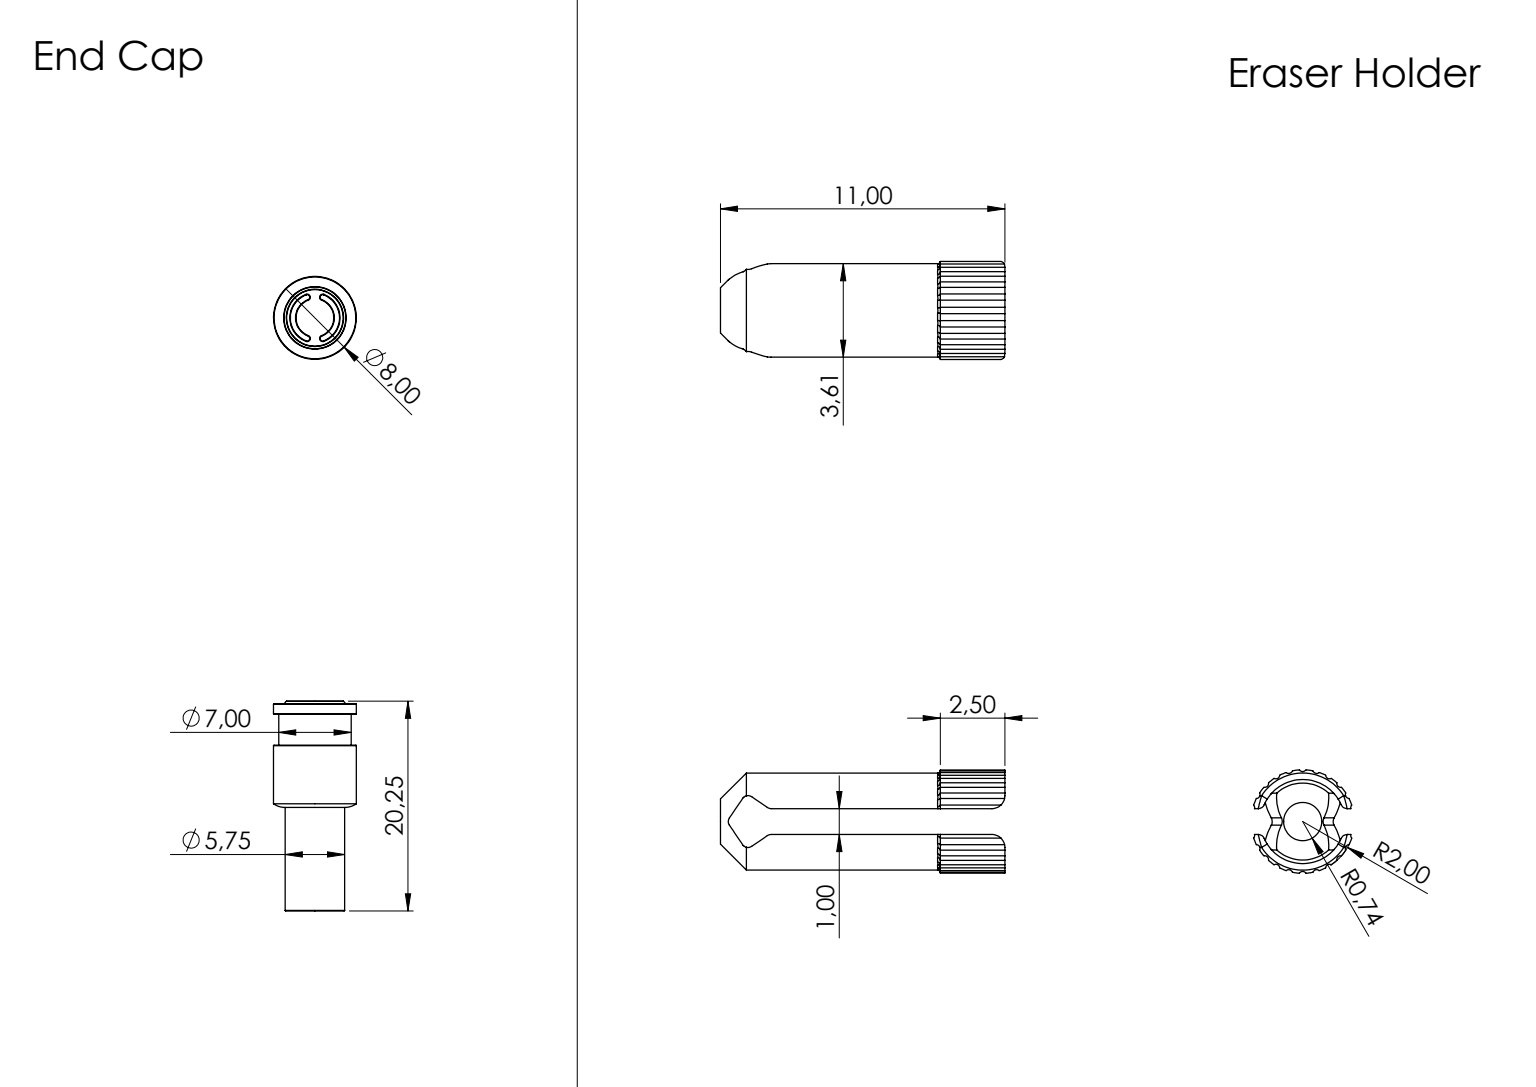
ISO-10303-21;
HEADER;
FILE_DESCRIPTION (('STEP AP214'),
    '1' );
FILE_NAME ('End Cap.step',
    '2026-10-06T14:00:01',
    ( '' ),
    ( '' ),
    'SwSTEP 2.0',
    'SolidWorks 2020',
    '' );
FILE_SCHEMA (( 'AUTOMOTIVE_DESIGN' ));
ENDSEC;

DATA;
#24=ORIENTED_EDGE ( 'NONE', *, *, #28945, .F. ) ;
#26=FACE_OUTER_BOUND ( 'NONE', #14344, .T. ) ;
#31=ORIENTED_EDGE ( 'NONE', *, *, #27047, .T. ) ;
#73=CARTESIAN_POINT ( 'NONE',  ( 63.50000000000004263, 0.7500000000000000000, 1.988246715072691018 ) ) ;
#80=DIRECTION ( 'NONE',  ( -1.000000000000000000, 0.000000000000000000, 1.047444401652940007E-14 ) ) ;
#85=( NAMED_UNIT ( * ) SI_UNIT ( $, .STERADIAN. ) SOLID_ANGLE_UNIT ( ) );
#109=EDGE_LOOP ( 'NONE', ( #31265, #1632, #31131, #2632 ) ) ;
#130=ORIENTED_EDGE ( 'NONE', *, *, #8388, .T. ) ;
#171=VERTEX_POINT ( 'NONE', #25293 ) ;
#187=FACE_OUTER_BOUND ( 'NONE', #28111, .T. ) ;
#235=ORIENTED_EDGE ( 'NONE', *, *, #4200, .F. ) ;
#258=CIRCLE ( 'NONE', #12381, 0.2999999999999999334 ) ;
#277=TOROIDAL_SURFACE ( 'NONE', #6855, 3.950000000000000178, 0.05000000000000000278 ) ;
#289=FACE_OUTER_BOUND ( 'NONE', #17501, .T. ) ;
#305=CIRCLE ( 'NONE', #30133, 0.05000000000000014849 ) ;
#318=AXIS2_PLACEMENT_3D ( 'NONE', #9279, #4194, #20999 ) ;
#319=ORIENTED_EDGE ( 'NONE', *, *, #23903, .T. ) ;
#326=ORIENTED_EDGE ( 'NONE', *, *, #1422, .T. ) ;
#340=CIRCLE ( 'NONE', #30668, 0.05000000000000007216 ) ;
#342=PLANE ( 'NONE',  #13632 ) ;
#352=DIRECTION ( 'NONE',  ( -1.000000000000000000, -0.000000000000000000, 1.047444401652940007E-14 ) ) ;
#365=AXIS2_PLACEMENT_3D ( 'NONE', #25779, #23413, #7408 ) ;
#369=ORIENTED_EDGE ( 'NONE', *, *, #19982, .T. ) ;
#372=ORIENTED_EDGE ( 'NONE', *, *, #29152, .T. ) ;
#391=( NAMED_UNIT ( * ) PLANE_ANGLE_UNIT ( ) SI_UNIT ( $, .RADIAN. ) );
#430=ORIENTED_EDGE ( 'NONE', *, *, #6181, .F. ) ;
#439=CARTESIAN_POINT ( 'NONE',  ( 69.20000000000005969, -0.7500000000000000000, 1.988246715072633508 ) ) ;
#454=DIRECTION ( 'NONE',  ( -1.000000000000000000, 0.000000000000000000, 1.047444401652940007E-14 ) ) ;
#460=EDGE_CURVE ( 'NONE', #25198, #24785, #24329, .T. ) ;
#474=ORIENTED_EDGE ( 'NONE', *, *, #7320, .T. ) ;
#479=DIRECTION ( 'NONE',  ( 1.000000000000000000, -0.000000000000000000, -1.047444401652940007E-14 ) ) ;
#486=APPLICATION_CONTEXT ( 'automotive_design' ) ;
#491=TOROIDAL_SURFACE ( 'NONE', #10107, 2.674999999999998934, 0.05000000000000000278 ) ;
#501=EDGE_CURVE ( 'NONE', #21780, #20962, #6621, .T. ) ;
#506=DIRECTION ( 'NONE',  ( 0.000000000000000000, -0.3529411764705882026, -0.9356455129756979794 ) ) ;
#512=PLANE ( 'NONE',  #27168 ) ;
#523=AXIS2_PLACEMENT_3D ( 'NONE', #6717, #4335, #11637 ) ;
#537=DIRECTION ( 'NONE',  ( 0.000000000000000000, 0.000000000000000000, -1.000000000000000000 ) ) ;
#590=VERTEX_POINT ( 'NONE', #30867 ) ;
#592=DIRECTION ( 'NONE',  ( 1.000000000000000000, -0.000000000000000000, -1.047444401652940007E-14 ) ) ;
#596=VERTEX_POINT ( 'NONE', #23754 ) ;
#602=EDGE_CURVE ( 'NONE', #9917, #10580, #19823, .T. ) ;
#617=FACE_OUTER_BOUND ( 'NONE', #26372, .T. ) ;
#662=DIRECTION ( 'NONE',  ( -1.000000000000000000, 0.000000000000000000, 1.047444401652940007E-14 ) ) ;
#666=ORIENTED_EDGE ( 'NONE', *, *, #5798, .T. ) ;
#670=EDGE_CURVE ( 'NONE', #23530, #30383, #28927, .T. ) ;
#679=DIRECTION ( 'NONE',  ( 1.000000000000000000, 0.000000000000000000, -1.047444401652940007E-14 ) ) ;
#690=DIRECTION ( 'NONE',  ( -1.000000000000000000, 0.000000000000000000, 1.047444401652940007E-14 ) ) ;
#696=ADVANCED_FACE ( 'NONE', ( #29416 ), #18309, .T. ) ;
#723=LINE ( 'NONE', #10382, #22147 ) ;
#738=EDGE_CURVE ( 'NONE', #5843, #8754, #4762, .T. ) ;
#757=CARTESIAN_POINT ( 'NONE',  ( 68.00000000000001421, 1.401298464324817071E-42, -7.122621931239992550E-13 ) ) ;
#763=VECTOR ( 'NONE', #13667, 1000.000000000000114 ) ;
#776=DIRECTION ( 'NONE',  ( 1.000000000000000000, -0.000000000000000000, -1.047444401652940007E-14 ) ) ;
#799=DIRECTION ( 'NONE',  ( 1.000000000000000000, 0.000000000000000000, -1.047444401652940007E-14 ) ) ;
#808=DIRECTION ( 'NONE',  ( 1.000000000000000000, -0.000000000000000000, -1.047444401652940007E-14 ) ) ;
#815=CIRCLE ( 'NONE', #18531, 0.2999999999999999334 ) ;
#824=DIRECTION ( 'NONE',  ( -1.000000000000000000, 0.000000000000000000, 1.047444401652940007E-14 ) ) ;
#859=EDGE_CURVE ( 'NONE', #27662, #23750, #12840, .T. ) ;
#865=VERTEX_POINT ( 'NONE', #10878 ) ;
#868=CLOSED_SHELL ( 'NONE', ( #3607, #31285, #19814, #2896, #11313, #1933, #16606, #2566, #11194, #9119, #8437, #4942, #20881, #10226, #9824, #19849, #13450, #13335, #9869, #14567, #23249, #23818, #19671, #16010, #18689, #8050, #28313, #23742, #25301, #4603, #23913, #2405, #3250, #16375, #22683, #11024, #14689, #29311, #10151, #2320, #31083, #28868, #9802, #29845, #22522, #28501, #27572, #16956, #21743, #3102, #20819, #24145, #21081, #696, #22329, #7299, #2322, #17235, #15972, #26956, #25336, #8923, #24762, #17568 ) ) ;
#899=TOROIDAL_SURFACE ( 'NONE', #1389, 1.824999999999999956, 0.05000000000000000278 ) ;
#913=EDGE_LOOP ( 'NONE', ( #29372, #10833, #15778, #13748, #18804, #24361, #21663, #28963, #6278, #30255, #1776, #13627, #28648, #7508, #21353, #15239 ) ) ;
#914=DIRECTION ( 'NONE',  ( -1.000000000000000000, 0.000000000000000000, 1.047444401652940007E-14 ) ) ;
#924=EDGE_LOOP ( 'NONE', ( #13849, #2269, #25709, #4752 ) ) ;
#937=TOROIDAL_SURFACE ( 'NONE', #5490, 3.950000000000000178, 0.05000000000000000278 ) ;
#1025=ORIENTED_EDGE ( 'NONE', *, *, #13535, .T. ) ;
#1027=CIRCLE ( 'NONE', #6586, 0.2999999999999999334 ) ;
#1078=EDGE_CURVE ( 'NONE', #25198, #6138, #25891, .T. ) ;
#1094=AXIS2_PLACEMENT_3D ( 'NONE', #17029, #80, #10049 ) ;
#1102=CARTESIAN_POINT ( 'NONE',  ( 67.99999999999998579, 1.401298464324817071E-42, -2.375000000000710543 ) ) ;
#1173=CARTESIAN_POINT ( 'NONE',  ( 68.00000000000000000, -0.6617647058823529216, -1.754335336830145975 ) ) ;
#1176=EDGE_LOOP ( 'NONE', ( #16382, #26534, #25910, #24778 ) ) ;
#1254=CARTESIAN_POINT ( 'NONE',  ( 68.05000000000006821, 4.898587196589419731E-16, 3.999999999999287237 ) ) ;
#1283=ORIENTED_EDGE ( 'NONE', *, *, #4003, .T. ) ;
#1296=AXIS2_PLACEMENT_3D ( 'NONE', #22942, #10594, #8211 ) ;
#1322=VECTOR ( 'NONE', #690, 1000.000000000000000 ) ;
#1330=ORIENTED_EDGE ( 'NONE', *, *, #14511, .F. ) ;
#1340=CARTESIAN_POINT ( 'NONE',  ( 60.67929986713514978, 1.401298464324817071E-42, -6.355819294205068152E-13 ) ) ;
#1361=TOROIDAL_SURFACE ( 'NONE', #10968, 0.3000000000000000444, 0.05000000000000000278 ) ;
#1385=VECTOR ( 'NONE', #24043, 1000.000000000000000 ) ;
#1389=AXIS2_PLACEMENT_3D ( 'NONE', #19677, #29454, #22353 ) ;
#1422=EDGE_CURVE ( 'NONE', #14417, #27508, #12555, .T. ) ;
#1434=EDGE_CURVE ( 'NONE', #12273, #27518, #6793, .T. ) ;
#1444=EDGE_LOOP ( 'NONE', ( #5295, #15394 ) ) ;
#1450=DIRECTION ( 'NONE',  ( 1.000000000000000000, -0.000000000000000000, -1.047444401652940007E-14 ) ) ;
#1517=EDGE_LOOP ( 'NONE', ( #10786, #26947 ) ) ;
#1554=DIRECTION ( 'NONE',  ( 0.000000000000000000, 0.000000000000000000, 1.000000000000000000 ) ) ;
#1566=DIRECTION ( 'NONE',  ( 1.000000000000000000, -0.000000000000000000, -1.047444401652940007E-14 ) ) ;
#1585=CARTESIAN_POINT ( 'NONE',  ( 67.99999999999998579, 3.214697847761800597E-16, -2.625000000000710987 ) ) ;
#1614=CARTESIAN_POINT ( 'NONE',  ( 63.50000000000000000, 0.7500000000000000000, -2.238246715074021953 ) ) ;
#1632=ORIENTED_EDGE ( 'NONE', *, *, #29506, .T. ) ;
#1669=EDGE_CURVE ( 'NONE', #12243, #22848, #26520, .T. ) ;
#1673=ORIENTED_EDGE ( 'NONE', *, *, #1078, .F. ) ;
#1683=CARTESIAN_POINT ( 'NONE',  ( 49.00000000000004263, -0.6617647058823530326, 1.754335336828920511 ) ) ;
#1692=VERTEX_POINT ( 'NONE', #27979 ) ;
#1728=DIRECTION ( 'NONE',  ( 1.040834085586084257E-14, 0.000000000000000000, 1.000000000000000000 ) ) ;
#1729=DIRECTION ( 'NONE',  ( -1.000000000000000000, -0.000000000000000000, 1.047444401652940007E-14 ) ) ;
#1752=VERTEX_POINT ( 'NONE', #10881 ) ;
#1766=EDGE_CURVE ( 'NONE', #1752, #14189, #12854, .T. ) ;
#1770=FACE_OUTER_BOUND ( 'NONE', #25402, .T. ) ;
#1775=DIRECTION ( 'NONE',  ( 0.000000000000000000, 0.000000000000000000, -1.000000000000000000 ) ) ;
#1776=ORIENTED_EDGE ( 'NONE', *, *, #6848, .T. ) ;
#1779=PLANE ( 'NONE',  #27597 ) ;
#1785=VERTEX_POINT ( 'NONE', #1980 ) ;
#1789=CARTESIAN_POINT ( 'NONE',  ( 69.24999999999998579, 3.823533025773894613E-16, -2.750000000000725198 ) ) ;
#1793=CARTESIAN_POINT ( 'NONE',  ( 68.00000000000004263, 0.8382352941176474115, 2.222158093316569438 ) ) ;
#1811=EDGE_CURVE ( 'NONE', #13465, #25040, #31059, .T. ) ;
#1853=CARTESIAN_POINT ( 'NONE',  ( 69.25000000000004263, -0.7500000000000000000, 1.988246715072630844 ) ) ;
#1869=CARTESIAN_POINT ( 'NONE',  ( 49.00000000000002132, 1.401298464324817071E-42, -5.132477568099407673E-13 ) ) ;
#1890=ORIENTED_EDGE ( 'NONE', *, *, #27079, .T. ) ;
#1912=CARTESIAN_POINT ( 'NONE',  ( 65.00000000000007105, 1.401298464324817071E-42, 3.499999999999319211 ) ) ;
#1933=ADVANCED_FACE ( 'NONE', ( #21468 ), #23872, .T. ) ;
#1963=EDGE_LOOP ( 'NONE', ( #10035, #26095, #29334, #18935, #7350, #21515, #2912 ) ) ;
#1966=EDGE_LOOP ( 'NONE', ( #11467, #21378, #11264, #28038 ) ) ;
#1976=VERTEX_POINT ( 'NONE', #17476 ) ;
#1980=CARTESIAN_POINT ( 'NONE',  ( 69.00000000000000000, 4.155057991226904698E-16, -3.020710678119368886 ) ) ;
#1984=CARTESIAN_POINT ( 'NONE',  ( 68.00000000000000000, 0.5000000000000000000, -1.988246715074070581 ) ) ;
#2001=DIRECTION ( 'NONE',  ( 1.000000000000000000, 0.000000000000000000, -1.047444401652940007E-14 ) ) ;
#2052=EDGE_CURVE ( 'NONE', #14020, #27339, #18813, .T. ) ;
#2071=CARTESIAN_POINT ( 'NONE',  ( 69.20000000000001705, 0.6617647058823536987, -1.754335336830159076 ) ) ;
#2089=DIRECTION ( 'NONE',  ( -1.047444401652940007E-14, 0.000000000000000000, -1.000000000000000000 ) ) ;
#2133=FACE_OUTER_BOUND ( 'NONE', #19427, .T. ) ;
#2155=EDGE_CURVE ( 'NONE', #20739, #26219, #22857, .T. ) ;
#2160=ORIENTED_EDGE ( 'NONE', *, *, #24446, .T. ) ;
#2166=DIRECTION ( 'NONE',  ( 1.000000000000000000, 0.000000000000000000, -1.047444401652940007E-14 ) ) ;
#2205=CARTESIAN_POINT ( 'NONE',  ( 49.00000000000000000, -0.6617647058823530326, -1.754335336829947023 ) ) ;
#2229=ORIENTED_EDGE ( 'NONE', *, *, #25840, .T. ) ;
#2256=DIRECTION ( 'NONE',  ( 1.000000000000000000, 0.000000000000000000, -1.047444401652940007E-14 ) ) ;
#2269=ORIENTED_EDGE ( 'NONE', *, *, #25539, .T. ) ;
#2275=DIRECTION ( 'NONE',  ( 1.000000000000000000, -0.000000000000000000, -1.047444401652940007E-14 ) ) ;
#2284=DIRECTION ( 'NONE',  ( -1.144559819201192819E-14, 0.000000000000000000, -1.000000000000000000 ) ) ;
#2296=DIRECTION ( 'NONE',  ( 1.047444401652940007E-14, 0.000000000000000000, 1.000000000000000000 ) ) ;
#2310=CARTESIAN_POINT ( 'NONE',  ( 69.20000000000001705, -0.7500000000000000000, -1.988246715074082793 ) ) ;
#2320=ADVANCED_FACE ( 'NONE', ( #26791 ), #10012, .F. ) ;
#2322=ADVANCED_FACE ( 'NONE', ( #16982 ), #491, .T. ) ;
#2327=DIRECTION ( 'NONE',  ( -1.000000000000000000, 0.000000000000000000, 1.047444401652940007E-14 ) ) ;
#2328=CIRCLE ( 'NONE', #6366, 3.500000000000000000 ) ;
#2329=CIRCLE ( 'NONE', #22049, 0.2500000000000002220 ) ;
#2343=ORIENTED_EDGE ( 'NONE', *, *, #19355, .F. ) ;
#2361=VECTOR ( 'NONE', #20954, 1000.000000000000000 ) ;
#2376=AXIS2_PLACEMENT_3D ( 'NONE', #4697, #2327, #21679 ) ;
#2377=TOROIDAL_SURFACE ( 'NONE', #10980, 0.3000000000000000444, 0.05000000000000000278 ) ;
#2390=CIRCLE ( 'NONE', #20103, 0.05000000000000012768 ) ;
#2405=ADVANCED_FACE ( 'NONE', ( #23799, #187, #22044 ), #342, .T. ) ;
#2482=DIRECTION ( 'NONE',  ( -1.047444401652940007E-14, 0.000000000000000000, -1.000000000000000000 ) ) ;
#2521=STYLED_ITEM ( 'NONE', ( #12068 ), #28934 ) ;
#2558=ORIENTED_EDGE ( 'NONE', *, *, #15305, .T. ) ;
#2565=SURFACE_STYLE_FILL_AREA ( #28995 ) ;
#2566=ADVANCED_FACE ( 'NONE', ( #11393 ), #11623, .T. ) ;
#2568=DIRECTION ( 'NONE',  ( -1.000000000000000000, 0.000000000000000000, 1.047444401652940007E-14 ) ) ;
#2591=DIRECTION ( 'NONE',  ( 1.047444401652940007E-14, 0.000000000000000000, 1.000000000000000000 ) ) ;
#2597=ORIENTED_EDGE ( 'NONE', *, *, #12546, .T. ) ;
#2632=ORIENTED_EDGE ( 'NONE', *, *, #11598, .F. ) ;
#2633=DIRECTION ( 'NONE',  ( 9.654113257610060303E-15, 0.000000000000000000, 1.000000000000000000 ) ) ;
#2689=DIRECTION ( 'NONE',  ( 0.000000000000000000, 0.000000000000000000, -1.000000000000000000 ) ) ;
#2696=CIRCLE ( 'NONE', #21934, 0.05000000000000012768 ) ;
#2699=CIRCLE ( 'NONE', #20918, 3.950000000000000178 ) ;
#2708=CARTESIAN_POINT ( 'NONE',  ( 69.25000000000000000, -0.7500000000000000000, -1.988246715074083681 ) ) ;
#2716=CIRCLE ( 'NONE', #6762, 2.374999999999998668 ) ;
#2745=VERTEX_POINT ( 'NONE', #14391 ) ;
#2748=LINE ( 'NONE', #17317, #16749 ) ;
#2761=EDGE_CURVE ( 'NONE', #21492, #16699, #6541, .T. ) ;
#2763=ORIENTED_EDGE ( 'NONE', *, *, #24226, .F. ) ;
#2779=AXIS2_PLACEMENT_3D ( 'NONE', #22887, #11146, #6100 ) ;
#2788=DIRECTION ( 'NONE',  ( -1.000000000000000000, 0.000000000000000000, 1.047444401652940007E-14 ) ) ;
#2792=CARTESIAN_POINT ( 'NONE',  ( 68.00000000000004263, 0.5000000000000000000, 1.988246715072646387 ) ) ;
#2797=AXIS2_PLACEMENT_3D ( 'NONE', #16721, #25731, #14318 ) ;
#2798=EDGE_LOOP ( 'NONE', ( #5175, #12651, #13298, #19894 ) ) ;
#2799=DIRECTION ( 'NONE',  ( 1.040834085586084257E-14, 0.000000000000000000, 1.000000000000000000 ) ) ;
#2811=DIRECTION ( 'NONE',  ( -1.000000000000000000, -0.000000000000000000, 1.047444401652940007E-14 ) ) ;
#2815=AXIS2_PLACEMENT_3D ( 'NONE', #16284, #25927, #4230 ) ;
#2873=CIRCLE ( 'NONE', #17554, 2.985355339059319046 ) ;
#2896=ADVANCED_FACE ( 'NONE', ( #3432 ), #10591, .F. ) ;
#2911=DIRECTION ( 'NONE',  ( -1.000000000000000000, -0.000000000000000000, 1.047444401652940007E-14 ) ) ;
#2912=ORIENTED_EDGE ( 'NONE', *, *, #24728, .T. ) ;
#2922=SURFACE_STYLE_FILL_AREA ( #16873 ) ;
#2956=PRODUCT_DEFINITION ( 'UNKNOWN', '', #17169, #15507 ) ;
#2979=LINE ( 'NONE', #9792, #28702 ) ;
#2982=DIRECTION ( 'NONE',  ( 0.000000000000000000, 0.000000000000000000, -1.000000000000000000 ) ) ;
#3000=CARTESIAN_POINT ( 'NONE',  ( 49.00000000000004974, 1.401298464324817071E-42, 2.824999999999485922 ) ) ;
#3035=CARTESIAN_POINT ( 'NONE',  ( 69.25000000000001421, 4.557543281186736018E-17, -7.253552481446610839E-13 ) ) ;
#3049=DIRECTION ( 'NONE',  ( 0.000000000000000000, -1.224646799147343593E-16, 1.000000000000000000 ) ) ;
#3050=CARTESIAN_POINT ( 'NONE',  ( 68.00000000000002842, 1.401298464324817071E-42, -7.122621931239993559E-13 ) ) ;
#3064=VERTEX_POINT ( 'NONE', #13827 ) ;
#3094=ORIENTED_EDGE ( 'NONE', *, *, #7320, .F. ) ;
#3102=ADVANCED_FACE ( 'NONE', ( #16561 ), #9433, .T. ) ;
#3117=EDGE_CURVE ( 'NONE', #24431, #23786, #25591, .T. ) ;
#3223=EDGE_CURVE ( 'NONE', #171, #9260, #10953, .T. ) ;
#3232=AXIS2_PLACEMENT_3D ( 'NONE', #3050, #824, #8112 ) ;
#3250=ADVANCED_FACE ( 'NONE', ( #5739 ), #28634, .T. ) ;
#3256=AXIS2_PLACEMENT_3D ( 'NONE', #9828, #19494, #5079 ) ;
#3264=AXIS2_PLACEMENT_3D ( 'NONE', #8768, #18933, #21165 ) ;
#3265=LINE ( 'NONE', #22761, #28622 ) ;
#3270=AXIS2_PLACEMENT_3D ( 'NONE', #13221, #20700, #30471 ) ;
#3274=DIRECTION ( 'NONE',  ( -1.047444401652940007E-14, 0.000000000000000000, -1.000000000000000000 ) ) ;
#3276=CARTESIAN_POINT ( 'NONE',  ( 69.20000000000001705, -0.5000000000000000000, -1.988246715074081017 ) ) ;
#3295=CARTESIAN_POINT ( 'NONE',  ( 65.00000000000002842, 1.401298464324817071E-42, -6.808388610744111684E-13 ) ) ;
#3304=CIRCLE ( 'NONE', #9890, 3.020710678118645909 ) ;
#3317=CIRCLE ( 'NONE', #2815, 4.000000000000000000 ) ;
#3382=VECTOR ( 'NONE', #15294, 1000.000000000000000 ) ;
#3387=DIRECTION ( 'NONE',  ( 1.047444401652940007E-14, 0.000000000000000000, 1.000000000000000000 ) ) ;
#3432=FACE_OUTER_BOUND ( 'NONE', #1176, .T. ) ;
#3433=CARTESIAN_POINT ( 'NONE',  ( 69.00000000000005684, 1.401298464324817071E-42, 3.949999999999278089 ) ) ;
#3442=CARTESIAN_POINT ( 'NONE',  ( 68.95000000000007390, 1.401298464324817071E-42, 3.949999999999278089 ) ) ;
#3506=DIRECTION ( 'NONE',  ( 1.000000000000000000, 0.000000000000000000, -1.047444401652940007E-14 ) ) ;
#3517=FACE_OUTER_BOUND ( 'NONE', #4297, .T. ) ;
#3522=DIRECTION ( 'NONE',  ( 1.168655815394902336E-14, 0.000000000000000000, 1.000000000000000000 ) ) ;
#3526=EDGE_LOOP ( 'NONE', ( #19588, #28740, #24, #29141 ) ) ;
#3530=DIRECTION ( 'NONE',  ( -3.198643159535995633E-15, -0.9356455129756995337, -0.3529411764705844834 ) ) ;
#3531=DIRECTION ( 'NONE',  ( 1.000000000000000000, 0.000000000000000000, -1.047444401652940007E-14 ) ) ;
#3543=DIRECTION ( 'NONE',  ( 1.000000000000000000, 0.000000000000000000, -8.673617379884989994E-15 ) ) ;
#3548=CARTESIAN_POINT ( 'NONE',  ( 49.05000000000002558, 1.401298464324817071E-42, -5.137714790107672405E-13 ) ) ;
#3607=ADVANCED_FACE ( 'NONE', ( #24484 ), #22978, .T. ) ;
#3713=ORIENTED_EDGE ( 'NONE', *, *, #27923, .F. ) ;
#3719=DIRECTION ( 'NONE',  ( -1.000000000000000000, 0.000000000000000000, 1.047444401652940007E-14 ) ) ;
#3738=ORIENTED_EDGE ( 'NONE', *, *, #8941, .F. ) ;
#3789=ORIENTED_EDGE ( 'NONE', *, *, #20362, .F. ) ;
#3797=CARTESIAN_POINT ( 'NONE',  ( 69.20000000000001705, 0.4500000000000000111, -1.988246715074080573 ) ) ;
#3811=DIRECTION ( 'NONE',  ( 1.000000000000000000, 0.000000000000000000, -1.047444401652940007E-14 ) ) ;
#3817=VERTEX_POINT ( 'NONE', #30595 ) ;
#3836=AXIS2_PLACEMENT_3D ( 'NONE', #5703, #8382, #22493 ) ;
#3844=EDGE_CURVE ( 'NONE', #14189, #1752, #2699, .T. ) ;
#3847=EDGE_CURVE ( 'NONE', #26053, #4809, #15343, .T. ) ;
#3856=VECTOR ( 'NONE', #15914, 1000.000000000000000 ) ;
#3869=AXIS2_PLACEMENT_3D ( 'NONE', #11567, #28818, #21242 ) ;
#3883=CIRCLE ( 'NONE', #21613, 0.2500000000000000000 ) ;
#3920=CIRCLE ( 'NONE', #27677, 1.874999999999998668 ) ;
#3988=ORIENTED_EDGE ( 'NONE', *, *, #18972, .F. ) ;
#4003=EDGE_CURVE ( 'NONE', #8546, #4409, #24941, .T. ) ;
#4006=DIRECTION ( 'NONE',  ( -1.040834085586084257E-14, 0.000000000000000000, -1.000000000000000000 ) ) ;
#4014=DIRECTION ( 'NONE',  ( 1.000000000000000000, -0.000000000000000000, -1.047444401652940007E-14 ) ) ;
#4016=ORIENTED_EDGE ( 'NONE', *, *, #22796, .F. ) ;
#4021=ORIENTED_EDGE ( 'NONE', *, *, #26922, .T. ) ;
#4023=LINE ( 'NONE', #1789, #763 ) ;
#4042=CIRCLE ( 'NONE', #19235, 0.05000000000000012768 ) ;
#4065=CARTESIAN_POINT ( 'NONE',  ( 58.99999999999999289, 4.286263797015737088E-16, -3.000000000000618172 ) ) ;
#4097=VERTEX_POINT ( 'NONE', #22985 ) ;
#4142=EDGE_CURVE ( 'NONE', #13465, #11082, #28489, .T. ) ;
#4158=CARTESIAN_POINT ( 'NONE',  ( 69.25000000000004263, -0.4500000000000000111, 1.988246715072632620 ) ) ;
#4175=CARTESIAN_POINT ( 'NONE',  ( 64.95000000000001705, 1.401298464324817071E-42, -6.803151388735846952E-13 ) ) ;
#4194=DIRECTION ( 'NONE',  ( 0.000000000000000000, -1.000000000000000000, -0.000000000000000000 ) ) ;
#4200=EDGE_CURVE ( 'NONE', #8754, #8529, #16324, .T. ) ;
#4230=DIRECTION ( 'NONE',  ( -1.040834085586084257E-14, 0.000000000000000000, -1.000000000000000000 ) ) ;
#4263=DIRECTION ( 'NONE',  ( 1.000000000000000000, 0.000000000000000000, -1.047444401652940007E-14 ) ) ;
#4297=EDGE_LOOP ( 'NONE', ( #27696, #15667, #12138, #14102 ) ) ;
#4314=CIRCLE ( 'NONE', #15443, 4.000000000000000000 ) ;
#4335=DIRECTION ( 'NONE',  ( -1.000000000000000000, 0.000000000000000000, 1.047444401652940007E-14 ) ) ;
#4339=ORIENTED_EDGE ( 'NONE', *, *, #3223, .T. ) ;
#4386=AXIS2_PLACEMENT_3D ( 'NONE', #20623, #10633, #30085 ) ;
#4409=VERTEX_POINT ( 'NONE', #14725 ) ;
#4451=EDGE_LOOP ( 'NONE', ( #20168, #369, #23422, #5115 ) ) ;
#4471=CARTESIAN_POINT ( 'NONE',  ( 65.00000000000002842, 1.401298464324817071E-42, -6.808388610744111684E-13 ) ) ;
#4472=CARTESIAN_POINT ( 'NONE',  ( 69.25000000000001421, 4.557543281186736018E-17, -7.253552481446610839E-13 ) ) ;
#4522=FACE_OUTER_BOUND ( 'NONE', #25805, .T. ) ;
#4554=DIRECTION ( 'NONE',  ( 1.000000000000000000, -0.000000000000000000, -1.047444401652940007E-14 ) ) ;
#4565=CARTESIAN_POINT ( 'NONE',  ( 63.50000000000002842, 1.401298464324817071E-42, -6.651271950496169736E-13 ) ) ;
#4566=VERTEX_POINT ( 'NONE', #7905 ) ;
#4579=CYLINDRICAL_SURFACE ( 'NONE', #25145, 4.000000000000000000 ) ;
#4595=DIRECTION ( 'NONE',  ( 0.000000000000000000, 0.000000000000000000, -1.000000000000000000 ) ) ;
#4603=ADVANCED_FACE ( 'NONE', ( #27697 ), #12797, .T. ) ;
#4641=AXIS2_PLACEMENT_3D ( 'NONE', #6535, #25844, #25994 ) ;
#4659=ORIENTED_EDGE ( 'NONE', *, *, #9443, .F. ) ;
#4681=DIRECTION ( 'NONE',  ( 1.000000000000000000, -0.000000000000000000, -1.047444401652940007E-14 ) ) ;
#4686=CARTESIAN_POINT ( 'NONE',  ( 69.25000000000001421, 1.401298464324817071E-42, -7.253552481446610839E-13 ) ) ;
#4697=CARTESIAN_POINT ( 'NONE',  ( 59.35000000000002984, 1.401298464324817071E-42, -6.216582523810200043E-13 ) ) ;
#4722=AXIS2_PLACEMENT_3D ( 'NONE', #17774, #30404, #22841 ) ;
#4752=ORIENTED_EDGE ( 'NONE', *, *, #29152, .F. ) ;
#4762=CIRCLE ( 'NONE', #19449, 2.624999999999998668 ) ;
#4778=AXIS2_PLACEMENT_3D ( 'NONE', #7989, #19867, #24604 ) ;
#4801=VERTEX_POINT ( 'NONE', #15636 ) ;
#4809=VERTEX_POINT ( 'NONE', #3276 ) ;
#4824=DIRECTION ( 'NONE',  ( -1.000000000000000000, 0.000000000000000000, 1.047444401652940007E-14 ) ) ;
#4825=CARTESIAN_POINT ( 'NONE',  ( 69.23535533905938166, 4.557543281186736018E-17, 2.764644660939941101 ) ) ;
#4840=DIRECTION ( 'NONE',  ( 1.000000000000000000, -0.000000000000000000, -1.047444401652940007E-14 ) ) ;
#4843=CARTESIAN_POINT ( 'NONE',  ( 68.00000000000000000, 0.7500000000000000000, -1.988246715074068582 ) ) ;
#4861=AXIS2_PLACEMENT_3D ( 'NONE', #18898, #23956, #16205 ) ;
#4880=CARTESIAN_POINT ( 'NONE',  ( 68.00000000000001421, 5.529431079676072613E-15, -7.122621931239992550E-13 ) ) ;
#4919=ORIENTED_EDGE ( 'NONE', *, *, #6181, .T. ) ;
#4928=( NAMED_UNIT ( * ) SI_UNIT ( $, .STERADIAN. ) SOLID_ANGLE_UNIT ( ) );
#4932=CIRCLE ( 'NONE', #25130, 2.874999999999999112 ) ;
#4942=ADVANCED_FACE ( 'NONE', ( #12268 ), #9903, .F. ) ;
#4959=FACE_OUTER_BOUND ( 'NONE', #16370, .T. ) ;
#4974=CARTESIAN_POINT ( 'NONE',  ( 65.00000000000007105, 4.867971026610729436E-16, 3.949999999999319389 ) ) ;
#4978=AXIS2_PLACEMENT_3D ( 'NONE', #73, #2275, #11940 ) ;
#4982=DIRECTION ( 'NONE',  ( 0.000000000000000000, 0.000000000000000000, -1.000000000000000000 ) ) ;
#5031=ORIENTED_EDGE ( 'NONE', *, *, #19144, .F. ) ;
#5051=CARTESIAN_POINT ( 'NONE',  ( 69.20000000000003126, 5.529431079676072613E-15, -7.248315259438346108E-13 ) ) ;
#5052=AXIS2_PLACEMENT_3D ( 'NONE', #23868, #7386, #19431 ) ;
#5079=DIRECTION ( 'NONE',  ( -7.401486830834377462E-15, 0.000000000000000000, -1.000000000000000000 ) ) ;
#5115=ORIENTED_EDGE ( 'NONE', *, *, #5759, .F. ) ;
#5127=ORIENTED_EDGE ( 'NONE', *, *, #24333, .F. ) ;
#5131=FACE_OUTER_BOUND ( 'NONE', #8472, .T. ) ;
#5138=CARTESIAN_POINT ( 'NONE',  ( 69.20000000000000284, -0.8558823529411765385, -2.268940368966790189 ) ) ;
#5175=ORIENTED_EDGE ( 'NONE', *, *, #18929, .F. ) ;
#5180=DIRECTION ( 'NONE',  ( 1.000000000000000000, 0.000000000000000000, -1.047444401652940007E-14 ) ) ;
#5218=CARTESIAN_POINT ( 'NONE',  ( 69.20000000000004547, 0.7500000000000000000, 1.988246715072631732 ) ) ;
#5226=ORIENTED_EDGE ( 'NONE', *, *, #18865, .F. ) ;
#5256=CARTESIAN_POINT ( 'NONE',  ( 68.94999999999998863, 4.837354856632045057E-16, -3.950000000000722711 ) ) ;
#5295=ORIENTED_EDGE ( 'NONE', *, *, #14044, .T. ) ;
#5306=CIRCLE ( 'NONE', #8845, 0.2999999999999999334 ) ;
#5348=CIRCLE ( 'NONE', #13423, 1.679509022399086948 ) ;
#5362=CIRCLE ( 'NONE', #24578, 0.05000000000000012768 ) ;
#5368=DIRECTION ( 'NONE',  ( -1.047444401652940007E-14, 0.000000000000000000, -1.000000000000000000 ) ) ;
#5381=AXIS2_PLACEMENT_3D ( 'NONE', #12530, #352, #26937 ) ;
#5385=DIRECTION ( 'NONE',  ( 1.168655815394902336E-14, 5.329070518200751394E-15, 1.000000000000000000 ) ) ;
#5411=DIRECTION ( 'NONE',  ( 1.047444401652940007E-14, 0.000000000000000000, 1.000000000000000000 ) ) ;
#5416=DIRECTION ( 'NONE',  ( -1.000000000000000000, 0.000000000000000000, 1.047444401652940007E-14 ) ) ;
#5436=AXIS2_PLACEMENT_3D ( 'NONE', #29883, #15788, #29727 ) ;
#5443=EDGE_LOOP ( 'NONE', ( #6142, #21561, #27785, #16734 ) ) ;
#5444=DIRECTION ( 'NONE',  ( 1.000000000000000000, -0.000000000000000000, -1.047444401652940007E-14 ) ) ;
#5456=CARTESIAN_POINT ( 'NONE',  ( 69.20000000000001705, -0.6441176470588234615, -1.707553061181373621 ) ) ;
#5465=ORIENTED_EDGE ( 'NONE', *, *, #5759, .T. ) ;
#5473=AXIS2_PLACEMENT_3D ( 'NONE', #13711, #30194, #10722 ) ;
#5490=AXIS2_PLACEMENT_3D ( 'NONE', #5911, #13312, #25370 ) ;
#5521=CARTESIAN_POINT ( 'NONE',  ( 69.20000000000003126, 1.401298464324817071E-42, -7.248315259438346108E-13 ) ) ;
#5589=CARTESIAN_POINT ( 'NONE',  ( 69.25000000000000000, -0.6441176470588234615, -1.707553061181374066 ) ) ;
#5640=LINE ( 'NONE', #17989, #3382 ) ;
#5646=LINE ( 'NONE', #23523, #3856 ) ;
#5672=LINE ( 'NONE', #24506, #9916 ) ;
#5703=CARTESIAN_POINT ( 'NONE',  ( 68.00000000000001421, 1.401298464324817071E-42, -7.122621931239992550E-13 ) ) ;
#5713=EDGE_CURVE ( 'NONE', #596, #25040, #2979, .T. ) ;
#5739=FACE_OUTER_BOUND ( 'NONE', #8033, .T. ) ;
#5759=EDGE_CURVE ( 'NONE', #25198, #27301, #19312, .T. ) ;
#5765=CARTESIAN_POINT ( 'NONE',  ( 59.00000000000006395, 4.898587196589412829E-16, 3.999999999999382716 ) ) ;
#5798=EDGE_CURVE ( 'NONE', #8746, #596, #3920, .T. ) ;
#5818=VERTEX_POINT ( 'NONE', #9952 ) ;
#5843=VERTEX_POINT ( 'NONE', #30025 ) ;
#5851=VECTOR ( 'NONE', #21513, 1000.000000000000000 ) ;
#5880=CIRCLE ( 'NONE', #9442, 0.2500000000000000000 ) ;
#5884=CARTESIAN_POINT ( 'NONE',  ( 69.25000000000000000, -0.7500000000000000000, -2.288246715074081283 ) ) ;
#5901=VERTEX_POINT ( 'NONE', #18014 ) ;
#5903=DIRECTION ( 'NONE',  ( -1.000000000000000000, -0.000000000000000000, 1.047444401652940007E-14 ) ) ;
#5911=CARTESIAN_POINT ( 'NONE',  ( 68.05000000000002558, 1.401298464324817071E-42, -7.127859153248258291E-13 ) ) ;
#5935=EDGE_CURVE ( 'NONE', #20739, #23786, #31228, .T. ) ;
#5937=ORIENTED_EDGE ( 'NONE', *, *, #18457, .T. ) ;
#5953=VERTEX_POINT ( 'NONE', #22780 ) ;
#5983=EDGE_LOOP ( 'NONE', ( #2229, #9730, #15226, #28249 ) ) ;
#5990=FACE_OUTER_BOUND ( 'NONE', #1966, .T. ) ;
#5993=DIRECTION ( 'NONE',  ( -9.654113257610060303E-15, 0.000000000000000000, -1.000000000000000000 ) ) ;
#6004=AXIS2_PLACEMENT_3D ( 'NONE', #21933, #27119, #10042 ) ;
#6014=ORIENTED_EDGE ( 'NONE', *, *, #19790, .T. ) ;
#6016=ORIENTED_EDGE ( 'NONE', *, *, #602, .F. ) ;
#6017=UNCERTAINTY_MEASURE_WITH_UNIT (LENGTH_MEASURE( 1.000000000000000082E-05 ), #6831, 'distance_accuracy_value', 'NONE');
#6023=EDGE_LOOP ( 'NONE', ( #3988, #12062, #15679, #11566, #29583, #12414, #7163, #22036 ) ) ;
#6049=DIRECTION ( 'NONE',  ( 1.003947306782822575E-14, 0.000000000000000000, 1.000000000000000000 ) ) ;
#6055=CARTESIAN_POINT ( 'NONE',  ( 68.95000000000003126, 1.401298464324817071E-42, -7.222129149397022450E-13 ) ) ;
#6062=FACE_OUTER_BOUND ( 'NONE', #18360, .T. ) ;
#6095=CARTESIAN_POINT ( 'NONE',  ( 64.99999999999998579, 4.286263797015736595E-16, -3.500000000000680789 ) ) ;
#6100=DIRECTION ( 'NONE',  ( 0.000000000000000000, 0.000000000000000000, -1.000000000000000000 ) ) ;
#6108=VERTEX_POINT ( 'NONE', #4065 ) ;
#6138=VERTEX_POINT ( 'NONE', #20864 ) ;
#6142=ORIENTED_EDGE ( 'NONE', *, *, #27708, .F. ) ;
#6158=EDGE_CURVE ( 'NONE', #9761, #29519, #8484, .T. ) ;
#6181=EDGE_CURVE ( 'NONE', #3817, #2745, #22155, .T. ) ;
#6204=EDGE_LOOP ( 'NONE', ( #235, #8965, #1890, #9902 ) ) ;
#6212=ORIENTED_EDGE ( 'NONE', *, *, #20691, .F. ) ;
#6241=CARTESIAN_POINT ( 'NONE',  ( 59.00000000000002132, 1.401298464324817071E-42, -6.179921969752347932E-13 ) ) ;
#6248=EDGE_LOOP ( 'NONE', ( #30369, #13520, #8307, #27484 ) ) ;
#6278=ORIENTED_EDGE ( 'NONE', *, *, #12527, .F. ) ;
#6290=EDGE_CURVE ( 'NONE', #9260, #18734, #19135, .T. ) ;
#6292=LINE ( 'NONE', #1683, #13720 ) ;
#6306=DIRECTION ( 'NONE',  ( 0.000000000000000000, 0.000000000000000000, -1.000000000000000000 ) ) ;
#6314=VERTEX_POINT ( 'NONE', #15606 ) ;
#6335=DIRECTION ( 'NONE',  ( 0.000000000000000000, 1.000000000000000000, -8.673617379884030739E-15 ) ) ;
#6347=DIRECTION ( 'NONE',  ( -9.654113257610060303E-15, 0.000000000000000000, -1.000000000000000000 ) ) ;
#6353=ORIENTED_EDGE ( 'NONE', *, *, #21694, .F. ) ;
#6366=AXIS2_PLACEMENT_3D ( 'NONE', #11355, #21044, #16429 ) ;
#6379=COLOUR_RGB ( '', 0.72549020, 0.75294118, 0.79215686) ;
#6392=AXIS2_PLACEMENT_3D ( 'NONE', #12568, #17654, #21801 ) ;
#6400=CIRCLE ( 'NONE', #318, 0.05000000000000012768 ) ;
#6405=CIRCLE ( 'NONE', #24108, 0.05000000000000014849 ) ;
#6416=CARTESIAN_POINT ( 'NONE',  ( 69.20000000000004547, -0.6617647058823530326, 1.754335336828708902 ) ) ;
#6435=CIRCLE ( 'NONE', #25111, 0.05000000000000012768 ) ;
#6436=ORIENTED_EDGE ( 'NONE', *, *, #9419, .F. ) ;
#6451=ORIENTED_EDGE ( 'NONE', *, *, #17555, .F. ) ;
#6461=DIRECTION ( 'NONE',  ( -1.000000000000000000, 0.000000000000000000, 1.047444401652940007E-14 ) ) ;
#6498=DIRECTION ( 'NONE',  ( 0.000000000000000000, 0.000000000000000000, -1.000000000000000000 ) ) ;
#6522=EDGE_LOOP ( 'NONE', ( #5031, #9393, #7409, #12142 ) ) ;
#6535=CARTESIAN_POINT ( 'NONE',  ( 68.00000000000004263, -0.7500000000000000000, 1.988246715072645943 ) ) ;
#6541=CIRCLE ( 'NONE', #12114, 2.374999999999998668 ) ;
#6557=DIRECTION ( 'NONE',  ( -1.047444401652940007E-14, 0.000000000000000000, -1.000000000000000000 ) ) ;
#6586=AXIS2_PLACEMENT_3D ( 'NONE', #12108, #13988, #7200 ) ;
#6621=CIRCLE ( 'NONE', #3836, 2.374999999999998668 ) ;
#6641=DIRECTION ( 'NONE',  ( 1.003947306782822575E-14, 0.000000000000000000, 1.000000000000000000 ) ) ;
#6687=DIRECTION ( 'NONE',  ( -1.282749433769087582E-30, 1.000000000000000000, -1.224646799147353207E-16 ) ) ;
#6710=CARTESIAN_POINT ( 'NONE',  ( 69.20000000000000284, -0.8382352941176473005, -2.222158093318006067 ) ) ;
#6717=CARTESIAN_POINT ( 'NONE',  ( 49.05000000000002558, 1.401298464324817071E-42, -5.137714790107672405E-13 ) ) ;
#6735=CARTESIAN_POINT ( 'NONE',  ( 67.99999999999997158, 1.401298464324817071E-42, -4.000000000000712319 ) ) ;
#6754=LINE ( 'NONE', #21671, #14045 ) ;
#6762=AXIS2_PLACEMENT_3D ( 'NONE', #10644, #662, #3522 ) ;
#6776=CARTESIAN_POINT ( 'NONE',  ( 68.00000000000000000, 0.8382352941176474115, -2.222158093317993632 ) ) ;
#6779=AXIS2_PLACEMENT_3D ( 'NONE', #12653, #20286, #10905 ) ;
#6793=CIRCLE ( 'NONE', #18945, 0.2999999999999999334 ) ;
#6796=CARTESIAN_POINT ( 'NONE',  ( 69.23535533905935324, 4.557543281186736018E-17, -7.252018534634969470E-13 ) ) ;
#6803=AXIS2_PLACEMENT_3D ( 'NONE', #19590, #4840, #9292 ) ;
#6814=DIRECTION ( 'NONE',  ( -1.000000000000000000, 0.000000000000000000, 1.047444401652940007E-14 ) ) ;
#6820=CIRCLE ( 'NONE', #24510, 0.2500000000000000000 ) ;
#6827=DIRECTION ( 'NONE',  ( -1.000000000000000000, -0.000000000000000000, 1.047444401652940007E-14 ) ) ;
#6831=( LENGTH_UNIT ( ) NAMED_UNIT ( * ) SI_UNIT ( .MILLI., .METRE. ) );
#6837=PRODUCT_DEFINITION_SHAPE ( 'NONE', 'NONE',  #2956 ) ;
#6842=DIRECTION ( 'NONE',  ( -1.000000000000000000, 0.000000000000000000, 1.047444401652940007E-14 ) ) ;
#6848=EDGE_CURVE ( 'NONE', #21838, #596, #7587, .T. ) ;
#6850=CYLINDRICAL_SURFACE ( 'NONE', #4861, 0.2500000000000002220 ) ;
#6855=AXIS2_PLACEMENT_3D ( 'NONE', #15685, #28009, #11227 ) ;
#6866=DIRECTION ( 'NONE',  ( 1.000000000000000000, -0.000000000000000000, -1.047444401652940007E-14 ) ) ;
#6873=AXIS2_PLACEMENT_3D ( 'NONE', #21591, #9560, #14430 ) ;
#6905=AXIS2_PLACEMENT_3D ( 'NONE', #31304, #4554, #21972 ) ;
#6927=CIRCLE ( 'NONE', #20581, 2.764644660940665855 ) ;
#6935=CARTESIAN_POINT ( 'NONE',  ( 68.00000000000001421, 1.401298464324817071E-42, -7.122621931239992550E-13 ) ) ;
#6970=DIRECTION ( 'NONE',  ( 1.037591611799212092E-14, 0.000000000000000000, 1.000000000000000000 ) ) ;
#7010=CARTESIAN_POINT ( 'NONE',  ( 69.00000000000001421, 4.557543281186736018E-17, -7.227366371405287181E-13 ) ) ;
#7015=DIRECTION ( 'NONE',  ( 1.000000000000000000, 0.000000000000000000, -1.047444401652940007E-14 ) ) ;
#7035=DIRECTION ( 'NONE',  ( -1.000000000000000000, 0.000000000000000000, 1.047444401652940007E-14 ) ) ;
#7062=CYLINDRICAL_SURFACE ( 'NONE', #17557, 4.000000000000000000 ) ;
#7092=DIRECTION ( 'NONE',  ( -1.000000000000000000, 0.000000000000000000, 1.047444401652940007E-14 ) ) ;
#7141=DIRECTION ( 'NONE',  ( 1.000000000000000000, -0.000000000000000000, -1.047444401652940007E-14 ) ) ;
#7160=( NAMED_UNIT ( * ) PLANE_ANGLE_UNIT ( ) SI_UNIT ( $, .RADIAN. ) );
#7163=ORIENTED_EDGE ( 'NONE', *, *, #19184, .T. ) ;
#7180=ORIENTED_EDGE ( 'NONE', *, *, #15305, .F. ) ;
#7199=DIRECTION ( 'NONE',  ( -1.000000000000000000, 0.000000000000000000, 1.047444401652940007E-14 ) ) ;
#7200=DIRECTION ( 'NONE',  ( 0.000000000000000000, 0.000000000000000000, -1.000000000000000000 ) ) ;
#7206=ORIENTED_EDGE ( 'NONE', *, *, #18972, .T. ) ;
#7209=EDGE_CURVE ( 'NONE', #31227, #21014, #22285, .T. ) ;
#7226=FACE_OUTER_BOUND ( 'NONE', #5983, .T. ) ;
#7232=EDGE_CURVE ( 'NONE', #4566, #6138, #20260, .T. ) ;
#7235=DIRECTION ( 'NONE',  ( 0.000000000000000000, -1.224646799147343593E-16, 1.000000000000000000 ) ) ;
#7238=DIRECTION ( 'NONE',  ( 1.000000000000000000, 0.000000000000000000, -1.047444401652940007E-14 ) ) ;
#7244=CARTESIAN_POINT ( 'NONE',  ( 64.95000000000001705, 1.401298464324817071E-42, -6.803151388735846952E-13 ) ) ;
#7249=ORIENTED_EDGE ( 'NONE', *, *, #28162, .T. ) ;
#7283=CARTESIAN_POINT ( 'NONE',  ( 68.00000000000002842, 1.401298464324817071E-42, -7.122621931239993559E-13 ) ) ;
#7299=ADVANCED_FACE ( 'NONE', ( #19250 ), #27304, .T. ) ;
#7309=ORIENTED_EDGE ( 'NONE', *, *, #30775, .T. ) ;
#7314=CARTESIAN_POINT ( 'NONE',  ( 49.00000000000004263, 0.7500000000000000000, 1.988246715072845561 ) ) ;
#7320=EDGE_CURVE ( 'NONE', #11082, #4097, #1027, .T. ) ;
#7325=EDGE_LOOP ( 'NONE', ( #18337, #30496, #30400, #25685 ) ) ;
#7334=DIRECTION ( 'NONE',  ( 9.912705577010325352E-15, 0.000000000000000000, 1.000000000000000000 ) ) ;
#7340=EDGE_LOOP ( 'NONE', ( #30787, #319, #5465, #11322 ) ) ;
#7350=ORIENTED_EDGE ( 'NONE', *, *, #10583, .T. ) ;
#7362=DIRECTION ( 'NONE',  ( 0.000000000000000000, 0.3529411764705882026, 0.9356455129756979794 ) ) ;
#7379=AXIS2_PLACEMENT_3D ( 'NONE', #14315, #23985, #2284 ) ;
#7386=DIRECTION ( 'NONE',  ( 1.000000000000000000, -0.000000000000000000, -1.047444401652940007E-14 ) ) ;
#7395=DIRECTION ( 'NONE',  ( 1.000000000000000000, -0.000000000000000000, -1.047444401652940007E-14 ) ) ;
#7402=STYLED_ITEM ( 'NONE', ( #9744 ), #25849 ) ;
#7408=DIRECTION ( 'NONE',  ( 0.000000000000000000, -1.224646799147353207E-16, 1.000000000000000000 ) ) ;
#7409=ORIENTED_EDGE ( 'NONE', *, *, #20691, .T. ) ;
#7420=AXIS2_PLACEMENT_3D ( 'NONE', #3442, #28243, #13082 ) ;
#7487=AXIS2_PLACEMENT_3D ( 'NONE', #30027, #8343, #5993 ) ;
#7497=DIRECTION ( 'NONE',  ( 1.000000000000000000, 0.000000000000000000, -1.047444401652940007E-14 ) ) ;
#7508=ORIENTED_EDGE ( 'NONE', *, *, #6290, .T. ) ;
#7513=EDGE_CURVE ( 'NONE', #20962, #21492, #2748, .T. ) ;
#7518=CARTESIAN_POINT ( 'NONE',  ( 63.50000000000000000, 3.214697847761892795E-16, -2.625000000000663913 ) ) ;
#7541=ORIENTED_EDGE ( 'NONE', *, *, #25840, .F. ) ;
#7542=VERTEX_POINT ( 'NONE', #4974 ) ;
#7557=( GEOMETRIC_REPRESENTATION_CONTEXT ( 3 ) GLOBAL_UNCERTAINTY_ASSIGNED_CONTEXT ( ( #25318 ) ) GLOBAL_UNIT_ASSIGNED_CONTEXT ( ( #9836, #7160, #4928 ) ) REPRESENTATION_CONTEXT ( 'NONE', 'WORKASPACE' ) );
#7558=TOROIDAL_SURFACE ( 'NONE', #28276, 2.729289321881338548, 0.05000000000000000278 ) ;
#7585=DIRECTION ( 'NONE',  ( -1.040834085586084257E-14, 0.000000000000000000, -1.000000000000000000 ) ) ;
#7587=CIRCLE ( 'NONE', #5052, 0.2499999999999997780 ) ;
#7616=DIRECTION ( 'NONE',  ( 1.000000000000000000, 0.000000000000000000, -1.047444401652940007E-14 ) ) ;
#7642=DIRECTION ( 'NONE',  ( -1.000000000000000000, 0.000000000000000000, 1.047444401652940007E-14 ) ) ;
#7661=TOROIDAL_SURFACE ( 'NONE', #30401, 2.973495046502706796, 1.679509022399086948 ) ;
#7686=CARTESIAN_POINT ( 'NONE',  ( 49.05000000000002558, 1.401298464324817071E-42, -5.137714790107672405E-13 ) ) ;
#7701=DIRECTION ( 'NONE',  ( -1.000000000000000000, 0.000000000000000000, 1.047444401652940007E-14 ) ) ;
#7744=AXIS2_PLACEMENT_3D ( 'NONE', #4565, #21520, #26411 ) ;
#7766=CIRCLE ( 'NONE', #13805, 4.000000000000000000 ) ;
#7798=ORIENTED_EDGE ( 'NONE', *, *, #3847, .F. ) ;
#7849=DIRECTION ( 'NONE',  ( 0.000000000000000000, -1.224646799147353207E-16, 1.000000000000000000 ) ) ;
#7857=AXIS2_PLACEMENT_3D ( 'NONE', #11160, #15176, #20834 ) ;
#7864=DIRECTION ( 'NONE',  ( 1.189524669241238948E-14, 0.000000000000000000, 1.000000000000000000 ) ) ;
#7905=CARTESIAN_POINT ( 'NONE',  ( 68.00000000000007105, 1.401298464324817071E-42, 3.949999999999288303 ) ) ;
#7906=CARTESIAN_POINT ( 'NONE',  ( 69.25000000000004263, -0.8558823529411765385, 2.268940368965340237 ) ) ;
#7925=AXIS2_PLACEMENT_3D ( 'NONE', #24997, #479, #5385 ) ;
#7940=DIRECTION ( 'NONE',  ( 1.000000000000000000, 0.000000000000000000, -1.047444401652940007E-14 ) ) ;
#7974=CIRCLE ( 'NONE', #22132, 2.985355339059319046 ) ;
#7981=CARTESIAN_POINT ( 'NONE',  ( 49.00000000000004263, -0.7500000000000000000, 1.988246715072845117 ) ) ;
#7989=CARTESIAN_POINT ( 'NONE',  ( 59.00000000000002132, 1.401298464324817071E-42, -6.179921969752347932E-13 ) ) ;
#7994=LINE ( 'NONE', #5765, #23529 ) ;
#8033=EDGE_LOOP ( 'NONE', ( #4016, #22809, #130, #11595 ) ) ;
#8042=CARTESIAN_POINT ( 'NONE',  ( 68.95000000000007390, 4.898587196589412829E-16, 3.999999999999277467 ) ) ;
#8049=CIRCLE ( 'NONE', #17660, 0.2999999999999999334 ) ;
#8050=ADVANCED_FACE ( 'NONE', ( #12474 ), #12632, .F. ) ;
#8089=EDGE_CURVE ( 'NONE', #8546, #20739, #6292, .T. ) ;
#8091=DIRECTION ( 'NONE',  ( -1.047444401652940007E-14, 0.000000000000000000, -1.000000000000000000 ) ) ;
#8112=DIRECTION ( 'NONE',  ( 1.054009200593503061E-14, 0.000000000000000000, 1.000000000000000000 ) ) ;
#8125=CARTESIAN_POINT ( 'NONE',  ( 68.00000000000000000, -0.8382352941176474115, -2.222158093317993632 ) ) ;
#8133=CARTESIAN_POINT ( 'NONE',  ( 69.20000000000005969, -0.7500000000000000000, 1.988246715072633508 ) ) ;
#8142=ORIENTED_EDGE ( 'NONE', *, *, #18936, .T. ) ;
#8147=ORIENTED_EDGE ( 'NONE', *, *, #30619, .F. ) ;
#8159=ORIENTED_EDGE ( 'NONE', *, *, #4200, .T. ) ;
#8165=EDGE_CURVE ( 'NONE', #29519, #27339, #21861, .T. ) ;
#8198=ORIENTED_EDGE ( 'NONE', *, *, #9738, .F. ) ;
#8206=CARTESIAN_POINT ( 'NONE',  ( 69.00000000000001421, 1.401298464324817071E-42, -7.227366371405287181E-13 ) ) ;
#8211=DIRECTION ( 'NONE',  ( 1.047444401652940007E-14, 0.000000000000000000, 1.000000000000000000 ) ) ;
#8217=DIRECTION ( 'NONE',  ( 0.000000000000000000, 0.000000000000000000, -1.000000000000000000 ) ) ;
#8281=DIRECTION ( 'NONE',  ( 0.000000000000000000, -1.224646799147353207E-16, 1.000000000000000000 ) ) ;
#8293=DIRECTION ( 'NONE',  ( 0.000000000000000000, 0.000000000000000000, -1.000000000000000000 ) ) ;
#8305=ORIENTED_EDGE ( 'NONE', *, *, #22796, .T. ) ;
#8307=ORIENTED_EDGE ( 'NONE', *, *, #31164, .F. ) ;
#8325=EDGE_LOOP ( 'NONE', ( #16996, #8305, #8342, #13316 ) ) ;
#8342=ORIENTED_EDGE ( 'NONE', *, *, #26310, .T. ) ;
#8343=DIRECTION ( 'NONE',  ( 1.000000000000000000, 0.000000000000000000, -1.047444401652940007E-14 ) ) ;
#8355=CIRCLE ( 'NONE', #26050, 2.824999999999998845 ) ;
#8371=ORIENTED_EDGE ( 'NONE', *, *, #26125, .F. ) ;
#8382=DIRECTION ( 'NONE',  ( 1.000000000000000000, -0.000000000000000000, -1.047444401652940007E-14 ) ) ;
#8388=EDGE_CURVE ( 'NONE', #23530, #24915, #9922, .T. ) ;
#8421=EDGE_LOOP ( 'NONE', ( #13172, #2160, #8919, #666 ) ) ;
#8422=AXIS2_PLACEMENT_3D ( 'NONE', #26445, #30885, #19020 ) ;
#8424=DIRECTION ( 'NONE',  ( -1.047444401652940007E-14, 0.000000000000000000, -1.000000000000000000 ) ) ;
#8437=ADVANCED_FACE ( 'NONE', ( #12435 ), #7661, .T. ) ;
#8438=FACE_OUTER_BOUND ( 'NONE', #22028, .T. ) ;
#8456=CARTESIAN_POINT ( 'NONE',  ( 68.00000000000001421, 1.401298464324817071E-42, -7.122621931239992550E-13 ) ) ;
#8472=EDGE_LOOP ( 'NONE', ( #11284, #10964, #22415, #27231 ) ) ;
#8476=CIRCLE ( 'NONE', #10486, 0.2999999999999999334 ) ;
#8484=CIRCLE ( 'NONE', #21142, 2.424999999999998934 ) ;
#8517=DIRECTION ( 'NONE',  ( 1.000000000000000000, -0.000000000000000000, -1.047444401652940007E-14 ) ) ;
#8529=VERTEX_POINT ( 'NONE', #20833 ) ;
#8542=DIRECTION ( 'NONE',  ( 1.040834085586084257E-14, 0.000000000000000000, 1.000000000000000000 ) ) ;
#8546=VERTEX_POINT ( 'NONE', #6416 ) ;
#8575=CARTESIAN_POINT ( 'NONE',  ( 68.00000000000000000, -0.7500000000000000000, -1.988246715074070137 ) ) ;
#8605=CYLINDRICAL_SURFACE ( 'NONE', #29276, 0.2500000000000002220 ) ;
#8613=ORIENTED_EDGE ( 'NONE', *, *, #2052, .T. ) ;
#8673=DIRECTION ( 'NONE',  ( 1.000000000000000000, -0.000000000000000000, -1.047444401652940007E-14 ) ) ;
#8692=ORIENTED_EDGE ( 'NONE', *, *, #1811, .F. ) ;
#8746=VERTEX_POINT ( 'NONE', #17321 ) ;
#8754=VERTEX_POINT ( 'NONE', #7518 ) ;
#8768=CARTESIAN_POINT ( 'NONE',  ( 69.20000000000005969, 0.7500000000000000000, 1.988246715072633952 ) ) ;
#8813=AXIS2_PLACEMENT_3D ( 'NONE', #21486, #9754, #9615 ) ;
#8821=EDGE_CURVE ( 'NONE', #1692, #21492, #17289, .T. ) ;
#8836=CIRCLE ( 'NONE', #15943, 2.729289321881338548 ) ;
#8845=AXIS2_PLACEMENT_3D ( 'NONE', #2708, #19669, #24854 ) ;
#8856=AXIS2_PLACEMENT_3D ( 'NONE', #14679, #12447, #31308 ) ;
#8894=DIRECTION ( 'NONE',  ( 0.000000000000000000, 0.000000000000000000, -1.000000000000000000 ) ) ;
#8900=LINE ( 'NONE', #1614, #2361 ) ;
#8918=AXIS2_PLACEMENT_3D ( 'NONE', #10159, #27088, #5411 ) ;
#8919=ORIENTED_EDGE ( 'NONE', *, *, #14292, .T. ) ;
#8923=ADVANCED_FACE ( 'NONE', ( #11716, #16791 ), #19011, .T. ) ;
#8939=DIRECTION ( 'NONE',  ( -1.047444401652940007E-14, 0.000000000000000000, -1.000000000000000000 ) ) ;
#8941=EDGE_CURVE ( 'NONE', #12243, #29519, #6405, .T. ) ;
#8944=CARTESIAN_POINT ( 'NONE',  ( 59.34999999999998721, 1.401298464324817071E-42, -4.000000000000621725 ) ) ;
#8965=ORIENTED_EDGE ( 'NONE', *, *, #738, .F. ) ;
#9007=ORIENTED_EDGE ( 'NONE', *, *, #18178, .F. ) ;
#9018=AXIS2_PLACEMENT_3D ( 'NONE', #25987, #9060, #11596 ) ;
#9060=DIRECTION ( 'NONE',  ( 0.000000000000000000, 0.000000000000000000, 1.000000000000000000 ) ) ;
#9063=MECHANICAL_DESIGN_GEOMETRIC_PRESENTATION_REPRESENTATION('',(#2521),#7557);
#9071=CARTESIAN_POINT ( 'NONE',  ( 69.25000000000001421, 4.557543281186736018E-17, -7.253552481446610839E-13 ) ) ;
#9078=EDGE_CURVE ( 'NONE', #23530, #3064, #11474, .T. ) ;
#9110=CARTESIAN_POINT ( 'NONE',  ( 49.05000000000002558, 1.401298464324817071E-42, -5.137714790107672405E-13 ) ) ;
#9119=ADVANCED_FACE ( 'NONE', ( #25262 ), #1361, .T. ) ;
#9199=DIRECTION ( 'NONE',  ( 1.047444401652940007E-14, 8.673617379884032317E-15, 1.000000000000000000 ) ) ;
#9260=VERTEX_POINT ( 'NONE', #1984 ) ;
#9271=ORIENTED_EDGE ( 'NONE', *, *, #21690, .F. ) ;
#9279=CARTESIAN_POINT ( 'NONE',  ( 69.20000000000001705, 0.7500000000000000000, -2.288246715074080839 ) ) ;
#9292=DIRECTION ( 'NONE',  ( 0.000000000000000000, 0.000000000000000000, 1.000000000000000000 ) ) ;
#9335=AXIS2_PLACEMENT_3D ( 'NONE', #7244, #16909, #14825 ) ;
#9393=ORIENTED_EDGE ( 'NONE', *, *, #17901, .F. ) ;
#9400=EDGE_CURVE ( 'NONE', #8546, #14020, #16033, .T. ) ;
#9412=CIRCLE ( 'NONE', #25071, 0.05000000000000012768 ) ;
#9419=EDGE_CURVE ( 'NONE', #9917, #8529, #2390, .T. ) ;
#9433=TOROIDAL_SURFACE ( 'NONE', #27105, 0.3000000000000000444, 0.05000000000000000278 ) ;
#9442=AXIS2_PLACEMENT_3D ( 'NONE', #29666, #27295, #16043 ) ;
#9443=EDGE_CURVE ( 'NONE', #24785, #4566, #6435, .T. ) ;
#9489=EDGE_CURVE ( 'NONE', #1785, #10286, #23619, .T. ) ;
#9534=UNCERTAINTY_MEASURE_WITH_UNIT (LENGTH_MEASURE( 1.000000000000000082E-05 ), #24603, 'distance_accuracy_value', 'NONE');
#9540=ORIENTED_EDGE ( 'NONE', *, *, #31164, .T. ) ;
#9542=CIRCLE ( 'NONE', #27213, 2.374999999999998668 ) ;
#9548=ORIENTED_EDGE ( 'NONE', *, *, #30619, .T. ) ;
#9560=DIRECTION ( 'NONE',  ( -1.000000000000000000, 0.000000000000000000, 1.047444401652940007E-14 ) ) ;
#9584=ORIENTED_EDGE ( 'NONE', *, *, #14044, .F. ) ;
#9590=DIRECTION ( 'NONE',  ( 1.168655815394902336E-14, 0.000000000000000000, 1.000000000000000000 ) ) ;
#9615=DIRECTION ( 'NONE',  ( 0.000000000000000000, 0.000000000000000000, -1.000000000000000000 ) ) ;
#9623=DIRECTION ( 'NONE',  ( -1.144559819201192819E-14, 0.000000000000000000, -1.000000000000000000 ) ) ;
#9627=ORIENTED_EDGE ( 'NONE', *, *, #25003, .F. ) ;
#9629=CARTESIAN_POINT ( 'NONE',  ( 68.04999999999998295, 4.837354856632045057E-16, -3.950000000000713385 ) ) ;
#9678=LINE ( 'NONE', #28830, #18573 ) ;
#9708=AXIS2_PLACEMENT_3D ( 'NONE', #757, #454, #20102 ) ;
#9730=ORIENTED_EDGE ( 'NONE', *, *, #12546, .F. ) ;
#9738=EDGE_CURVE ( 'NONE', #590, #23750, #23801, .T. ) ;
#9744=PRESENTATION_STYLE_ASSIGNMENT (( #28898 ) ) ;
#9754=DIRECTION ( 'NONE',  ( 1.000000000000000000, -0.000000000000000000, -1.047444401652940007E-14 ) ) ;
#9761=VERTEX_POINT ( 'NONE', #29317 ) ;
#9762=DIRECTION ( 'NONE',  ( 1.000000000000000000, -0.000000000000000000, -1.047444401652940007E-14 ) ) ;
#9792=CARTESIAN_POINT ( 'NONE',  ( 49.00000000000004263, 0.6617647058823536987, 1.754335336828920955 ) ) ;
#9802=ADVANCED_FACE ( 'NONE', ( #29167 ), #899, .T. ) ;
#9803=DIRECTION ( 'NONE',  ( 1.000000000000000000, -0.000000000000000000, -1.047444401652940007E-14 ) ) ;
#9824=ADVANCED_FACE ( 'NONE', ( #19171 ), #14703, .F. ) ;
#9828=CARTESIAN_POINT ( 'NONE',  ( 69.20000000000003126, 3.252606517456513302E-16, -7.248315259438346108E-13 ) ) ;
#9836=( LENGTH_UNIT ( ) NAMED_UNIT ( * ) SI_UNIT ( .MILLI., .METRE. ) );
#9845=DIRECTION ( 'NONE',  ( 1.047444401652940007E-14, 0.000000000000000000, 1.000000000000000000 ) ) ;
#9858=AXIS2_PLACEMENT_3D ( 'NONE', #2310, #2001, #2482 ) ;
#9869=ADVANCED_FACE ( 'NONE', ( #28954 ), #4579, .T. ) ;
#9890=AXIS2_PLACEMENT_3D ( 'NONE', #7010, #2568, #16672 ) ;
#9898=AXIS2_PLACEMENT_3D ( 'NONE', #13756, #1729, #11397 ) ;
#9899=EDGE_CURVE ( 'NONE', #31290, #21780, #28705, .T. ) ;
#9902=ORIENTED_EDGE ( 'NONE', *, *, #10374, .T. ) ;
#9903=CYLINDRICAL_SURFACE ( 'NONE', #8813, 0.2500000000000002220 ) ;
#9916=VECTOR ( 'NONE', #9803, 1000.000000000000000 ) ;
#9917=VERTEX_POINT ( 'NONE', #21705 ) ;
#9922=LINE ( 'NONE', #26856, #28410 ) ;
#9926=AXIS2_PLACEMENT_3D ( 'NONE', #13643, #6687, #16348 ) ;
#9932=VECTOR ( 'NONE', #28865, 1000.000000000000000 ) ;
#9952=CARTESIAN_POINT ( 'NONE',  ( 59.00000000000000000, 1.401298464324817071E-42, -2.875000000000617284 ) ) ;
#9955=CARTESIAN_POINT ( 'NONE',  ( 69.25000000000000000, 0.8558823529411767606, -2.268940368966791965 ) ) ;
#9961=CARTESIAN_POINT ( 'NONE',  ( 63.50000000000002842, 1.401298464324817071E-42, -6.651271950496169736E-13 ) ) ;
#9969=ORIENTED_EDGE ( 'NONE', *, *, #26922, .F. ) ;
#9975=TOROIDAL_SURFACE ( 'NONE', #14002, 0.3000000000000000444, 0.05000000000000000278 ) ;
#9977=DIRECTION ( 'NONE',  ( -1.000000000000000000, -0.000000000000000000, 1.047444401652940007E-14 ) ) ;
#10002=SHAPE_REPRESENTATION_RELATIONSHIP ( 'NONE' , 'NONE' ,  #15725, #28934 ) ;
#10012=CYLINDRICAL_SURFACE ( 'NONE', #15163, 0.2500000000000000000 ) ;
#10035=ORIENTED_EDGE ( 'NONE', *, *, #1434, .T. ) ;
#10042=DIRECTION ( 'NONE',  ( 0.000000000000000000, 0.000000000000000000, -1.000000000000000000 ) ) ;
#10049=DIRECTION ( 'NONE',  ( 1.047444401652940007E-14, 0.000000000000000000, 1.000000000000000000 ) ) ;
#10076=AXIS2_PLACEMENT_3D ( 'NONE', #24938, #3719, #29858 ) ;
#10107=AXIS2_PLACEMENT_3D ( 'NONE', #31058, #6842, #9845 ) ;
#10151=ADVANCED_FACE ( 'NONE', ( #1770 ), #6850, .F. ) ;
#10159=CARTESIAN_POINT ( 'NONE',  ( 69.05000000000002558, 4.557543281186736018E-17, -7.232603593413552923E-13 ) ) ;
#10185=DIRECTION ( 'NONE',  ( 0.000000000000000000, 0.000000000000000000, -1.000000000000000000 ) ) ;
#10190=EDGE_CURVE ( 'NONE', #4801, #1976, #23657, .T. ) ;
#10226=ADVANCED_FACE ( 'NONE', ( #10310 ), #28655, .T. ) ;
#10234=DIRECTION ( 'NONE',  ( 0.000000000000000000, -1.000000000000000000, 0.000000000000000000 ) ) ;
#10244=ORIENTED_EDGE ( 'NONE', *, *, #1669, .T. ) ;
#10247=DIRECTION ( 'NONE',  ( -1.000000000000000000, 0.000000000000000000, 1.047444401652940007E-14 ) ) ;
#10253=CARTESIAN_POINT ( 'NONE',  ( 58.99999999999998579, 1.401298464324817071E-42, -4.000000000000617284 ) ) ;
#10286=VERTEX_POINT ( 'NONE', #17443 ) ;
#10288=EDGE_CURVE ( 'NONE', #12947, #15675, #25084, .T. ) ;
#10310=FACE_OUTER_BOUND ( 'NONE', #8325, .T. ) ;
#10324=EDGE_LOOP ( 'NONE', ( #21883, #12349, #26181, #26769 ) ) ;
#10325=ORIENTED_EDGE ( 'NONE', *, *, #9400, .F. ) ;
#10334=AXIS2_PLACEMENT_3D ( 'NONE', #5521, #14558, #12033 ) ;
#10345=SURFACE_SIDE_STYLE ('',( #2922 ) ) ;
#10374=EDGE_CURVE ( 'NONE', #6314, #8529, #11946, .T. ) ;
#10382=CARTESIAN_POINT ( 'NONE',  ( 63.50000000000004263, -0.8382352941176473005, 2.222158093316616068 ) ) ;
#10447=EDGE_LOOP ( 'NONE', ( #16398, #4021, #10661, #21143 ) ) ;
#10465=VECTOR ( 'NONE', #28353, 1000.000000000000000 ) ;
#10486=AXIS2_PLACEMENT_3D ( 'NONE', #24669, #2811, #2982 ) ;
#10501=CARTESIAN_POINT ( 'NONE',  ( 49.00000000000000000, 0.5000000000000000000, -1.988246715073869408 ) ) ;
#10521=TOROIDAL_SURFACE ( 'NONE', #28212, 2.973495046502706796, 1.679509022399086948 ) ;
#10537=ORIENTED_EDGE ( 'NONE', *, *, #28162, .F. ) ;
#10580=VERTEX_POINT ( 'NONE', #26763 ) ;
#10583=EDGE_CURVE ( 'NONE', #27339, #4409, #815, .T. ) ;
#10591=TOROIDAL_SURFACE ( 'NONE', #10076, 3.020710678118645909, 0.05000000000000000278 ) ;
#10594=DIRECTION ( 'NONE',  ( -1.000000000000000000, 0.000000000000000000, 1.047444401652940007E-14 ) ) ;
#10603=DIRECTION ( 'NONE',  ( -1.110223024625157329E-14, 0.000000000000000000, -1.000000000000000000 ) ) ;
#10633=DIRECTION ( 'NONE',  ( 1.000000000000000000, 0.000000000000000000, -1.047444401652940007E-14 ) ) ;
#10637=CARTESIAN_POINT ( 'NONE',  ( 49.00000000000002132, 1.401298464324817071E-42, -5.132477568099407673E-13 ) ) ;
#10639=CARTESIAN_POINT ( 'NONE',  ( 63.50000000000000000, 0.7500000000000000000, -1.988246715074021731 ) ) ;
#10644=CARTESIAN_POINT ( 'NONE',  ( 63.50000000000002842, 1.401298464324817071E-42, -6.651271950496169736E-13 ) ) ;
#10661=ORIENTED_EDGE ( 'NONE', *, *, #3847, .T. ) ;
#10674=DIRECTION ( 'NONE',  ( 1.000000000000000000, 0.000000000000000000, -1.047444401652940007E-14 ) ) ;
#10712=VERTEX_POINT ( 'NONE', #27988 ) ;
#10722=DIRECTION ( 'NONE',  ( 0.000000000000000000, 0.000000000000000000, -1.000000000000000000 ) ) ;
#10750=ORIENTED_EDGE ( 'NONE', *, *, #10288, .F. ) ;
#10760=DIRECTION ( 'NONE',  ( 1.000000000000000000, -0.000000000000000000, -1.047444401652940007E-14 ) ) ;
#10786=ORIENTED_EDGE ( 'NONE', *, *, #17782, .T. ) ;
#10804=CARTESIAN_POINT ( 'NONE',  ( 49.00000000000002132, 1.401298464324817071E-42, -5.132477568099407673E-13 ) ) ;
#10833=ORIENTED_EDGE ( 'NONE', *, *, #17555, .T. ) ;
#10878=CARTESIAN_POINT ( 'NONE',  ( 69.25000000000000000, 0.4500000000000000111, -1.988246715074081461 ) ) ;
#10881=CARTESIAN_POINT ( 'NONE',  ( 68.99999999999997158, 4.867971026610729436E-16, -3.950000000000722711 ) ) ;
#10904=ORIENTED_EDGE ( 'NONE', *, *, #9078, .F. ) ;
#10905=DIRECTION ( 'NONE',  ( -1.047444401652940007E-14, 0.000000000000000000, -1.000000000000000000 ) ) ;
#10953=LINE ( 'NONE', #10501, #21582 ) ;
#10964=ORIENTED_EDGE ( 'NONE', *, *, #9400, .T. ) ;
#10968=AXIS2_PLACEMENT_3D ( 'NONE', #25415, #23216, #8939 ) ;
#10974=EDGE_CURVE ( 'NONE', #27518, #9761, #8049, .T. ) ;
#10980=AXIS2_PLACEMENT_3D ( 'NONE', #439, #17542, #27194 ) ;
#10982=FACE_OUTER_BOUND ( 'NONE', #28895, .T. ) ;
#11024=ADVANCED_FACE ( 'NONE', ( #25706 ), #8605, .F. ) ;
#11028=ORIENTED_EDGE ( 'NONE', *, *, #26483, .F. ) ;
#11062=FACE_OUTER_BOUND ( 'NONE', #10447, .T. ) ;
#11082=VERTEX_POINT ( 'NONE', #31250 ) ;
#11088=CIRCLE ( 'NONE', #15137, 0.2500000000000002220 ) ;
#11139=ORIENTED_EDGE ( 'NONE', *, *, #18178, .T. ) ;
#11146=DIRECTION ( 'NONE',  ( 1.000000000000000000, -0.000000000000000000, -1.047444401652940007E-14 ) ) ;
#11160=CARTESIAN_POINT ( 'NONE',  ( 69.20000000000001705, 0.7500000000000000000, -1.988246715074081017 ) ) ;
#11173=EDGE_LOOP ( 'NONE', ( #9548, #1025 ) ) ;
#11194=ADVANCED_FACE ( 'NONE', ( #24877 ), #7558, .T. ) ;
#11227=DIRECTION ( 'NONE',  ( 1.047444401652940007E-14, 0.000000000000000000, 1.000000000000000000 ) ) ;
#11264=ORIENTED_EDGE ( 'NONE', *, *, #22994, .T. ) ;
#11284=ORIENTED_EDGE ( 'NONE', *, *, #8089, .F. ) ;
#11285=CIRCLE ( 'NONE', #12798, 0.05000000000000010686 ) ;
#11295=EDGE_LOOP ( 'NONE', ( #6014, #2597, #11666, #27365 ) ) ;
#11313=ADVANCED_FACE ( 'NONE', ( #25027 ), #17172, .T. ) ;
#11322=ORIENTED_EDGE ( 'NONE', *, *, #26476, .T. ) ;
#11355=CARTESIAN_POINT ( 'NONE',  ( 65.00000000000002842, 1.401298464324817071E-42, -6.808388610744111684E-13 ) ) ;
#11369=CARTESIAN_POINT ( 'NONE',  ( 69.20000000000000284, 4.557543281186736018E-17, -2.729289321882063302 ) ) ;
#11393=FACE_OUTER_BOUND ( 'NONE', #26489, .T. ) ;
#11397=DIRECTION ( 'NONE',  ( 0.000000000000000000, -7.228014483236697541E-16, -1.000000000000000000 ) ) ;
#11452=ORIENTED_EDGE ( 'NONE', *, *, #29823, .F. ) ;
#11455=AXIS2_PLACEMENT_3D ( 'NONE', #13864, #2166, #28926 ) ;
#11463=EDGE_LOOP ( 'NONE', ( #1283, #15001, #26197, #10325 ) ) ;
#11467=ORIENTED_EDGE ( 'NONE', *, *, #26483, .T. ) ;
#11474=CIRCLE ( 'NONE', #20603, 0.05000000000000012768 ) ;
#11535=CIRCLE ( 'NONE', #7420, 0.05000000000000012768 ) ;
#11539=DIRECTION ( 'NONE',  ( 1.000000000000000000, -0.000000000000000000, -1.047444401652940007E-14 ) ) ;
#11545=ORIENTED_EDGE ( 'NONE', *, *, #19499, .F. ) ;
#11566=ORIENTED_EDGE ( 'NONE', *, *, #501, .T. ) ;
#11567=CARTESIAN_POINT ( 'NONE',  ( 64.99999999999998579, 1.401298464324817071E-42, -3.500000000000680789 ) ) ;
#11595=ORIENTED_EDGE ( 'NONE', *, *, #15854, .T. ) ;
#11596=DIRECTION ( 'NONE',  ( 1.000000000000000000, 0.000000000000000000, 0.000000000000000000 ) ) ;
#11598=EDGE_CURVE ( 'NONE', #24542, #21838, #11088, .T. ) ;
#11609=CARTESIAN_POINT ( 'NONE',  ( 59.00000000000006395, 4.898587196589412829E-16, 3.999999999999382716 ) ) ;
#11623=TOROIDAL_SURFACE ( 'NONE', #19731, 0.3000000000000000444, 0.05000000000000000278 ) ;
#11627=FACE_OUTER_BOUND ( 'NONE', #23579, .T. ) ;
#11637=DIRECTION ( 'NONE',  ( 1.047444401652940007E-14, 0.000000000000000000, 1.000000000000000000 ) ) ;
#11666=ORIENTED_EDGE ( 'NONE', *, *, #17537, .F. ) ;
#11716=FACE_OUTER_BOUND ( 'NONE', #11173, .T. ) ;
#11727=PLANE ( 'NONE',  #8422 ) ;
#11732=EDGE_CURVE ( 'NONE', #30383, #21345, #4042, .T. ) ;
#11750=ORIENTED_EDGE ( 'NONE', *, *, #9489, .F. ) ;
#11783=ORIENTED_EDGE ( 'NONE', *, *, #27509, .F. ) ;
#11784=FACE_OUTER_BOUND ( 'NONE', #109, .T. ) ;
#11844=CARTESIAN_POINT ( 'NONE',  ( 68.00000000000004263, -0.8382352941176474115, 2.222158093316569438 ) ) ;
#11848=DIRECTION ( 'NONE',  ( 0.000000000000000000, -1.000000000000000000, -0.000000000000000000 ) ) ;
#11911=CARTESIAN_POINT ( 'NONE',  ( 68.95000000000003126, 1.401298464324817071E-42, -7.222129149397022450E-13 ) ) ;
#11940=DIRECTION ( 'NONE',  ( 0.000000000000000000, 0.000000000000000000, -1.000000000000000000 ) ) ;
#11946=CIRCLE ( 'NONE', #29145, 2.624999999999998668 ) ;
#11965=ORIENTED_EDGE ( 'NONE', *, *, #17328, .T. ) ;
#11970=( GEOMETRIC_REPRESENTATION_CONTEXT ( 3 ) GLOBAL_UNCERTAINTY_ASSIGNED_CONTEXT ( ( #9534 ) ) GLOBAL_UNIT_ASSIGNED_CONTEXT ( ( #24603, #391, #85 ) ) REPRESENTATION_CONTEXT ( 'NONE', 'WORKASPACE' ) );
#11997=CIRCLE ( 'NONE', #27680, 0.05000000000000002359 ) ;
#12029=DIRECTION ( 'NONE',  ( 1.168655815394902336E-14, 3.552713678800500929E-15, 1.000000000000000000 ) ) ;
#12033=DIRECTION ( 'NONE',  ( -1.168655815394902336E-14, 0.000000000000000000, -1.000000000000000000 ) ) ;
#12062=ORIENTED_EDGE ( 'NONE', *, *, #30957, .T. ) ;
#12068=PRESENTATION_STYLE_ASSIGNMENT (( #19358 ) ) ;
#12108=CARTESIAN_POINT ( 'NONE',  ( 69.25000000000004263, 0.7500000000000000000, 1.988246715072630844 ) ) ;
#12114=AXIS2_PLACEMENT_3D ( 'NONE', #24641, #22287, #23765 ) ;
#12138=ORIENTED_EDGE ( 'NONE', *, *, #3223, .F. ) ;
#12142=ORIENTED_EDGE ( 'NONE', *, *, #18936, .F. ) ;
#12188=EDGE_CURVE ( 'NONE', #25083, #20971, #20250, .T. ) ;
#12243=VERTEX_POINT ( 'NONE', #22115 ) ;
#12268=FACE_OUTER_BOUND ( 'NONE', #28081, .T. ) ;
#12273=VERTEX_POINT ( 'NONE', #31289 ) ;
#12291=LINE ( 'NONE', #19612, #5851 ) ;
#12315=CARTESIAN_POINT ( 'NONE',  ( 68.00000000000004263, 2.908536147974970122E-16, 2.374999999999286793 ) ) ;
#12349=ORIENTED_EDGE ( 'NONE', *, *, #9738, .T. ) ;
#12352=APPLICATION_CONTEXT ( 'automotive_design' ) ;
#12354=AXIS2_PLACEMENT_3D ( 'NONE', #19773, #29406, #17377 ) ;
#12373=AXIS2_PLACEMENT_3D ( 'NONE', #15855, #3530, #20640 ) ;
#12381=AXIS2_PLACEMENT_3D ( 'NONE', #28843, #6827, #16666 ) ;
#12403=AXIS2_PLACEMENT_3D ( 'NONE', #9110, #26361, #26036 ) ;
#12414=ORIENTED_EDGE ( 'NONE', *, *, #2761, .T. ) ;
#12419=DIRECTION ( 'NONE',  ( 1.168655815394902336E-14, 0.000000000000000000, 1.000000000000000000 ) ) ;
#12434=AXIS2_PLACEMENT_3D ( 'NONE', #13019, #23790, #28693 ) ;
#12435=FACE_OUTER_BOUND ( 'NONE', #23510, .T. ) ;
#12440=CIRCLE ( 'NONE', #19553, 0.05000000000000014849 ) ;
#12447=DIRECTION ( 'NONE',  ( -1.000000000000000000, 0.000000000000000000, 1.047444401652940007E-14 ) ) ;
#12455=EDGE_LOOP ( 'NONE', ( #7541, #1330, #27275, #6353 ) ) ;
#12474=FACE_OUTER_BOUND ( 'NONE', #6204, .T. ) ;
#12485=CIRCLE ( 'NONE', #365, 1.679509022399086948 ) ;
#12506=CARTESIAN_POINT ( 'NONE',  ( 69.20000000000001705, -0.7500000000000000000, -1.988246715074082793 ) ) ;
#12527=EDGE_CURVE ( 'NONE', #24542, #25083, #23131, .T. ) ;
#12530=CARTESIAN_POINT ( 'NONE',  ( 69.25000000000000000, 0.7500000000000000000, -1.988246715074081905 ) ) ;
#12536=CARTESIAN_POINT ( 'NONE',  ( 69.20000000000004547, -0.6441176470588234615, 1.707553061179923892 ) ) ;
#12538=DIRECTION ( 'NONE',  ( -1.047444401652940007E-14, 0.000000000000000000, -1.000000000000000000 ) ) ;
#12540=ORIENTED_EDGE ( 'NONE', *, *, #1078, .T. ) ;
#12546=EDGE_CURVE ( 'NONE', #4809, #10712, #27661, .T. ) ;
#12555=LINE ( 'NONE', #24590, #15396 ) ;
#12568=CARTESIAN_POINT ( 'NONE',  ( 69.20000000000004547, -0.7500000000000000000, 1.988246715072631732 ) ) ;
#12588=ORIENTED_EDGE ( 'NONE', *, *, #12188, .T. ) ;
#12607=ORIENTED_EDGE ( 'NONE', *, *, #17537, .T. ) ;
#12631=CARTESIAN_POINT ( 'NONE',  ( 69.20000000000004547, 0.6617647058823536987, 1.754335336828709346 ) ) ;
#12632=CYLINDRICAL_SURFACE ( 'NONE', #9708, 2.624999999999998668 ) ;
#12645=CARTESIAN_POINT ( 'NONE',  ( 68.00000000000004263, -0.6617647058823529216, 1.754335336828721337 ) ) ;
#12651=ORIENTED_EDGE ( 'NONE', *, *, #1811, .T. ) ;
#12653=CARTESIAN_POINT ( 'NONE',  ( 69.20000000000003126, 4.557543281186736018E-17, -7.248315259438346108E-13 ) ) ;
#12709=AXIS2_PLACEMENT_3D ( 'NONE', #1853, #15654, #25299 ) ;
#12716=DIRECTION ( 'NONE',  ( -3.696862594069216125E-15, 0.9356455129756975353, -0.3529411764705897570 ) ) ;
#12735=ORIENTED_EDGE ( 'NONE', *, *, #15624, .T. ) ;
#12758=ORIENTED_EDGE ( 'NONE', *, *, #24333, .T. ) ;
#12795=DIRECTION ( 'NONE',  ( 0.000000000000000000, -1.000000000000000000, 0.000000000000000000 ) ) ;
#12797=CYLINDRICAL_SURFACE ( 'NONE', #23202, 1.874999999999998668 ) ;
#12798=AXIS2_PLACEMENT_3D ( 'NONE', #30051, #29753, #20277 ) ;
#12838=DIRECTION ( 'NONE',  ( 1.282749433769087582E-30, 1.000000000000000000, 1.224646799147353207E-16 ) ) ;
#12840=CIRCLE ( 'NONE', #17928, 3.500000000000000000 ) ;
#12854=CIRCLE ( 'NONE', #14865, 3.950000000000000178 ) ;
#12919=CARTESIAN_POINT ( 'NONE',  ( 59.35000000000002984, 1.401298464324817071E-42, -6.216582523810200043E-13 ) ) ;
#12947=VERTEX_POINT ( 'NONE', #9955 ) ;
#12949=AXIS2_PLACEMENT_3D ( 'NONE', #5256, #12838, #3049 ) ;
#12959=EDGE_CURVE ( 'NONE', #21014, #11082, #8476, .T. ) ;
#12988=AXIS2_PLACEMENT_3D ( 'NONE', #16652, #13758, #4595 ) ;
#12993=FACE_OUTER_BOUND ( 'NONE', #11295, .T. ) ;
#13001=DIRECTION ( 'NONE',  ( 0.000000000000000000, -0.3529411764705844834, -0.9356455129756994227 ) ) ;
#13019=CARTESIAN_POINT ( 'NONE',  ( 69.25000000000001421, 4.557543281186736018E-17, -7.253552481446610839E-13 ) ) ;
#13063=DIRECTION ( 'NONE',  ( 1.054009200593503061E-14, 0.000000000000000000, 1.000000000000000000 ) ) ;
#13082=DIRECTION ( 'NONE',  ( 0.000000000000000000, 0.000000000000000000, -1.000000000000000000 ) ) ;
#13094=DIRECTION ( 'NONE',  ( 0.000000000000000000, -1.000000000000000000, -0.000000000000000000 ) ) ;
#13121=EDGE_LOOP ( 'NONE', ( #13201, #8159, #23204, #13412 ) ) ;
#13146=DIRECTION ( 'NONE',  ( 0.000000000000000000, 0.000000000000000000, -1.000000000000000000 ) ) ;
#13163=CARTESIAN_POINT ( 'NONE',  ( 69.00000000000001421, 4.557543281186736018E-17, -7.227366371405287181E-13 ) ) ;
#13172=ORIENTED_EDGE ( 'NONE', *, *, #5713, .T. ) ;
#13201=ORIENTED_EDGE ( 'NONE', *, *, #20997, .F. ) ;
#13203=CYLINDRICAL_SURFACE ( 'NONE', #2779, 0.2500000000000000000 ) ;
#13221=CARTESIAN_POINT ( 'NONE',  ( 64.95000000000001705, 1.401298464324817071E-42, -6.803151388735846952E-13 ) ) ;
#13254=PLANE ( 'NONE',  #1296 ) ;
#13266=ORIENTED_EDGE ( 'NONE', *, *, #8821, .T. ) ;
#13272=AXIS2_PLACEMENT_3D ( 'NONE', #21925, #26014, #13974 ) ;
#13298=ORIENTED_EDGE ( 'NONE', *, *, #5713, .F. ) ;
#13312=DIRECTION ( 'NONE',  ( -1.000000000000000000, 0.000000000000000000, 1.047444401652940007E-14 ) ) ;
#13316=ORIENTED_EDGE ( 'NONE', *, *, #8388, .F. ) ;
#13332=FACE_OUTER_BOUND ( 'NONE', #913, .T. ) ;
#13335=ADVANCED_FACE ( 'NONE', ( #10982 ), #25385, .T. ) ;
#13339=PLANE ( 'NONE',  #16325 ) ;
#13348=ORIENTED_EDGE ( 'NONE', *, *, #21902, .F. ) ;
#13362=CIRCLE ( 'NONE', #21022, 1.874999999999998668 ) ;
#13412=ORIENTED_EDGE ( 'NONE', *, *, #27079, .F. ) ;
#13414=ORIENTED_EDGE ( 'NONE', *, *, #26476, .F. ) ;
#13423=AXIS2_PLACEMENT_3D ( 'NONE', #27481, #10234, #20539 ) ;
#13433=AXIS2_PLACEMENT_3D ( 'NONE', #8575, #1450, #13468 ) ;
#13440=CYLINDRICAL_SURFACE ( 'NONE', #14521, 0.2499999999999997780 ) ;
#13446=DIRECTION ( 'NONE',  ( -3.696862594069160905E-15, 0.9356455129756995337, -0.3529411764705844834 ) ) ;
#13450=ADVANCED_FACE ( 'NONE', ( #8438 ), #18119, .T. ) ;
#13456=DIRECTION ( 'NONE',  ( 1.047444401652940007E-14, 0.000000000000000000, 1.000000000000000000 ) ) ;
#13459=ORIENTED_EDGE ( 'NONE', *, *, #28420, .T. ) ;
#13465=VERTEX_POINT ( 'NONE', #27590 ) ;
#13466=VECTOR ( 'NONE', #7238, 1000.000000000000000 ) ;
#13468=DIRECTION ( 'NONE',  ( 0.000000000000000000, 1.734723475976807094E-15, 1.000000000000000000 ) ) ;
#13477=DIRECTION ( 'NONE',  ( -1.000000000000000000, 0.000000000000000000, 8.673617379884989994E-15 ) ) ;
#13485=DIRECTION ( 'NONE',  ( 1.000000000000000000, -0.000000000000000000, -1.047444401652940007E-14 ) ) ;
#13518=ORIENTED_EDGE ( 'NONE', *, *, #15172, .T. ) ;
#13520=ORIENTED_EDGE ( 'NONE', *, *, #26125, .T. ) ;
#13535=EDGE_CURVE ( 'NONE', #7542, #14261, #26705, .T. ) ;
#13540=DIRECTION ( 'NONE',  ( -1.000000000000000000, 0.000000000000000000, 1.047444401652940007E-14 ) ) ;
#13609=ORIENTED_EDGE ( 'NONE', *, *, #18865, .T. ) ;
#13627=ORIENTED_EDGE ( 'NONE', *, *, #5798, .F. ) ;
#13632=AXIS2_PLACEMENT_3D ( 'NONE', #4472, #14125, #2089 ) ;
#13643=CARTESIAN_POINT ( 'NONE',  ( 64.95000000000005969, 4.837354856632045057E-16, 3.949999999999320277 ) ) ;
#13645=DIRECTION ( 'NONE',  ( 0.000000000000000000, -1.000000000000000000, 0.000000000000000000 ) ) ;
#13667=DIRECTION ( 'NONE',  ( -0.7071067811865561215, 8.659560562354918067E-17, -0.7071067811865388020 ) ) ;
#13671=DIRECTION ( 'NONE',  ( -1.040834085586084257E-14, 0.000000000000000000, -1.000000000000000000 ) ) ;
#13707=VERTEX_POINT ( 'NONE', #21395 ) ;
#13711=CARTESIAN_POINT ( 'NONE',  ( 69.20000000000001705, 0.7500000000000000000, -1.988246715074083237 ) ) ;
#13720=VECTOR ( 'NONE', #6461, 1000.000000000000000 ) ;
#13748=ORIENTED_EDGE ( 'NONE', *, *, #3117, .T. ) ;
#13756=CARTESIAN_POINT ( 'NONE',  ( 69.25000000000000000, 0.7500000000000000000, -1.988246715074084126 ) ) ;
#13758=DIRECTION ( 'NONE',  ( 0.000000000000000000, -1.000000000000000000, 0.000000000000000000 ) ) ;
#13791=CARTESIAN_POINT ( 'NONE',  ( 69.20000000000001705, -0.7500000000000000000, -2.288246715074080839 ) ) ;
#13798=DIRECTION ( 'NONE',  ( 1.054009200593503061E-14, 0.000000000000000000, 1.000000000000000000 ) ) ;
#13805=AXIS2_PLACEMENT_3D ( 'NONE', #12919, #914, #2799 ) ;
#13811=ORIENTED_EDGE ( 'NONE', *, *, #24504, .T. ) ;
#13827=CARTESIAN_POINT ( 'NONE',  ( 69.25000000000004263, 3.819818661513594083E-16, 2.729289321880612906 ) ) ;
#13849=ORIENTED_EDGE ( 'NONE', *, *, #1766, .F. ) ;
#13864=CARTESIAN_POINT ( 'NONE',  ( 69.25000000000001421, 4.557543281186736018E-17, -7.253552481446610839E-13 ) ) ;
#13874=CYLINDRICAL_SURFACE ( 'NONE', #21088, 2.874999999999999112 ) ;
#13903=ORIENTED_EDGE ( 'NONE', *, *, #30850, .T. ) ;
#13918=LINE ( 'NONE', #21091, #10465 ) ;
#13945=EDGE_LOOP ( 'NONE', ( #8371, #24737, #17010, #7798 ) ) ;
#13958=CARTESIAN_POINT ( 'NONE',  ( 69.25000000000000000, 0.7500000000000000000, -2.288246715074081283 ) ) ;
#13969=AXIS2_PLACEMENT_3D ( 'NONE', #10639, #29947, #19986 ) ;
#13974=DIRECTION ( 'NONE',  ( 1.040834085586084257E-14, 0.000000000000000000, 1.000000000000000000 ) ) ;
#13978=TOROIDAL_SURFACE ( 'NONE', #8918, 3.020710678118645909, 0.05000000000000000278 ) ;
#13984=EDGE_LOOP ( 'NONE', ( #27541, #8142 ) ) ;
#13988=DIRECTION ( 'NONE',  ( -1.000000000000000000, -0.000000000000000000, 1.047444401652940007E-14 ) ) ;
#14002=AXIS2_PLACEMENT_3D ( 'NONE', #21410, #23305, #21100 ) ;
#14020=VERTEX_POINT ( 'NONE', #30989 ) ;
#14034=AXIS2_PLACEMENT_3D ( 'NONE', #7686, #9762, #2633 ) ;
#14044=EDGE_CURVE ( 'NONE', #10580, #9917, #25604, .T. ) ;
#14045=VECTOR ( 'NONE', #26714, 1000.000000000000000 ) ;
#14089=DIRECTION ( 'NONE',  ( -1.000000000000000000, 0.000000000000000000, 1.047444401652940007E-14 ) ) ;
#14094=ORIENTED_EDGE ( 'NONE', *, *, #9419, .T. ) ;
#14102=ORIENTED_EDGE ( 'NONE', *, *, #16163, .T. ) ;
#14113=FILL_AREA_STYLE_COLOUR ( '', #16157 ) ;
#14124=DIRECTION ( 'NONE',  ( -1.054009200593503061E-14, 0.000000000000000000, -1.000000000000000000 ) ) ;
#14125=DIRECTION ( 'NONE',  ( 1.000000000000000000, 0.000000000000000000, -1.047444401652940007E-14 ) ) ;
#14151=ORIENTED_EDGE ( 'NONE', *, *, #4142, .T. ) ;
#14189=VERTEX_POINT ( 'NONE', #3433 ) ;
#14261=VERTEX_POINT ( 'NONE', #25266 ) ;
#14278=EDGE_LOOP ( 'NONE', ( #11750, #2763, #28179, #19625 ) ) ;
#14285=AXIS2_PLACEMENT_3D ( 'NONE', #14552, #31176, #7585 ) ;
#14292=EDGE_CURVE ( 'NONE', #28523, #8746, #5640, .T. ) ;
#14303=ORIENTED_EDGE ( 'NONE', *, *, #19865, .T. ) ;
#14315=CARTESIAN_POINT ( 'NONE',  ( 69.25000000000001421, 1.401298464324817071E-42, -7.253552481446610839E-13 ) ) ;
#14318=DIRECTION ( 'NONE',  ( 1.040834085586084257E-14, 0.000000000000000000, 1.000000000000000000 ) ) ;
#14344=EDGE_LOOP ( 'NONE', ( #10904, #11545, #19914, #9007 ) ) ;
#14349=AXIS2_PLACEMENT_3D ( 'NONE', #22609, #5180, #3274 ) ;
#14391=CARTESIAN_POINT ( 'NONE',  ( 49.05000000000005400, 3.520859547548703549E-16, 2.874999999999485745 ) ) ;
#14393=CARTESIAN_POINT ( 'NONE',  ( 68.00000000000000000, -0.7500000000000000000, -1.988246715074068582 ) ) ;
#14400=DIRECTION ( 'NONE',  ( -1.000000000000000000, 0.000000000000000000, 1.047444401652940007E-14 ) ) ;
#14417=VERTEX_POINT ( 'NONE', #8944 ) ;
#14430=DIRECTION ( 'NONE',  ( 1.047444401652940007E-14, 0.000000000000000000, 1.000000000000000000 ) ) ;
#14441=AXIS2_PLACEMENT_3D ( 'NONE', #7981, #24597, #4982 ) ;
#14453=EDGE_LOOP ( 'NONE', ( #27426, #7206, #12588, #21924, #10244, #23163, #22661, #3713 ) ) ;
#14511=EDGE_CURVE ( 'NONE', #4409, #23987, #26668, .T. ) ;
#14519=CYLINDRICAL_SURFACE ( 'NONE', #21082, 2.624999999999998668 ) ;
#14521=AXIS2_PLACEMENT_3D ( 'NONE', #17763, #22680, #13146 ) ;
#14552=CARTESIAN_POINT ( 'NONE',  ( 59.00000000000002132, 1.401298464324817071E-42, -6.179921969752347932E-13 ) ) ;
#14553=CARTESIAN_POINT ( 'NONE',  ( 59.00000000000002132, 1.401298464324817071E-42, -6.179921969752347932E-13 ) ) ;
#14558=DIRECTION ( 'NONE',  ( 1.000000000000000000, 0.000000000000000000, -1.047444401652940007E-14 ) ) ;
#14567=ADVANCED_FACE ( 'NONE', ( #28749 ), #7062, .T. ) ;
#14602=CARTESIAN_POINT ( 'NONE',  ( 69.01464466094070360, 4.557543281186736018E-17, -7.228900318216929560E-13 ) ) ;
#14642=FILL_AREA_STYLE_COLOUR ( '', #6379 ) ;
#14679=CARTESIAN_POINT ( 'NONE',  ( 49.00000000000002132, 1.401298464324817071E-42, -5.132477568099407673E-13 ) ) ;
#14689=ADVANCED_FACE ( 'NONE', ( #12993 ), #13440, .F. ) ;
#14703=CYLINDRICAL_SURFACE ( 'NONE', #17074, 2.374999999999998668 ) ;
#14712=AXIS2_PLACEMENT_3D ( 'NONE', #25001, #10760, #8542 ) ;
#14725=CARTESIAN_POINT ( 'NONE',  ( 69.25000000000004263, -0.6441176470588234615, 1.707553061179923448 ) ) ;
#14765=ORIENTED_EDGE ( 'NONE', *, *, #21414, .F. ) ;
#14817=TOROIDAL_SURFACE ( 'NONE', #20413, 2.424999999999998934, 0.05000000000000000278 ) ;
#14825=DIRECTION ( 'NONE',  ( -1.047444401652940007E-14, 0.000000000000000000, -1.000000000000000000 ) ) ;
#14865=AXIS2_PLACEMENT_3D ( 'NONE', #8206, #8517, #30359 ) ;
#14919=ORIENTED_EDGE ( 'NONE', *, *, #21365, .T. ) ;
#14938=DIRECTION ( 'NONE',  ( 3.696862594069201137E-15, -0.9356455129756980904, 0.3529411764705883137 ) ) ;
#14979=AXIS2_PLACEMENT_3D ( 'NONE', #3035, #22509, #19831 ) ;
#14981=CARTESIAN_POINT ( 'NONE',  ( 49.04999999999999716, 3.459627207591271682E-16, -2.825000000000512657 ) ) ;
#15001=ORIENTED_EDGE ( 'NONE', *, *, #10583, .F. ) ;
#15017=ORIENTED_EDGE ( 'NONE', *, *, #14292, .F. ) ;
#15035=DIRECTION ( 'NONE',  ( 1.000000000000000000, 0.000000000000000000, -1.047444401652940007E-14 ) ) ;
#15060=CARTESIAN_POINT ( 'NONE',  ( 68.00000000000004263, -0.7500000000000000000, 1.988246715072644166 ) ) ;
#15061=CARTESIAN_POINT ( 'NONE',  ( 59.34999999999999432, 4.286263797015737088E-16, -3.500000000000622169 ) ) ;
#15124=DIRECTION ( 'NONE',  ( 1.000000000000000000, -0.000000000000000000, -1.047444401652940007E-14 ) ) ;
#15137=AXIS2_PLACEMENT_3D ( 'NONE', #18359, #23116, #1554 ) ;
#15140=FACE_OUTER_BOUND ( 'NONE', #16829, .T. ) ;
#15153=EDGE_CURVE ( 'NONE', #22848, #31290, #3265, .T. ) ;
#15163=AXIS2_PLACEMENT_3D ( 'NONE', #7314, #26323, #24263 ) ;
#15172=EDGE_CURVE ( 'NONE', #4801, #28026, #5348, .T. ) ;
#15176=DIRECTION ( 'NONE',  ( 1.000000000000000000, 0.000000000000000000, -1.047444401652940007E-14 ) ) ;
#15226=ORIENTED_EDGE ( 'NONE', *, *, #31299, .F. ) ;
#15234=VERTEX_POINT ( 'NONE', #18787 ) ;
#15239=ORIENTED_EDGE ( 'NONE', *, *, #501, .F. ) ;
#15242=EDGE_LOOP ( 'NONE', ( #21147, #15853, #372, #13414 ) ) ;
#15270=AXIS2_PLACEMENT_3D ( 'NONE', #28013, #799, #29773 ) ;
#15294=DIRECTION ( 'NONE',  ( -1.000000000000000000, 0.000000000000000000, 1.047444401652940007E-14 ) ) ;
#15305=EDGE_CURVE ( 'NONE', #15675, #1692, #6400, .T. ) ;
#15341=DIRECTION ( 'NONE',  ( 0.000000000000000000, 0.000000000000000000, -1.000000000000000000 ) ) ;
#15343=CIRCLE ( 'NONE', #16879, 0.2499999999999997780 ) ;
#15394=ORIENTED_EDGE ( 'NONE', *, *, #602, .T. ) ;
#15395=FACE_OUTER_BOUND ( 'NONE', #21693, .T. ) ;
#15396=VECTOR ( 'NONE', #679, 1000.000000000000000 ) ;
#15405=CARTESIAN_POINT ( 'NONE',  ( 69.20000000000005969, -0.4500000000000000111, 1.988246715072633508 ) ) ;
#15438=CARTESIAN_POINT ( 'NONE',  ( 68.00000000000002842, 1.401298464324817071E-42, -7.122621931239993559E-13 ) ) ;
#15443=AXIS2_PLACEMENT_3D ( 'NONE', #4175, #20826, #13671 ) ;
#15448=CARTESIAN_POINT ( 'NONE',  ( 69.20000000000005969, 3.798169760107705143E-16, 2.729289321880613794 ) ) ;
#15452=CIRCLE ( 'NONE', #8856, 2.824999999999998845 ) ;
#15507=PRODUCT_DEFINITION_CONTEXT ( 'detailed design', #486, 'design' ) ;
#15555=CIRCLE ( 'NONE', #29209, 0.04999999999999969746 ) ;
#15576=DIRECTION ( 'NONE',  ( -9.654113257610060303E-15, 0.000000000000000000, -1.000000000000000000 ) ) ;
#15600=EDGE_CURVE ( 'NONE', #29622, #24431, #5880, .T. ) ;
#15606=CARTESIAN_POINT ( 'NONE',  ( 49.05000000000005400, 1.401298464324817071E-42, 2.624999999999484857 ) ) ;
#15607=ORIENTED_EDGE ( 'NONE', *, *, #16608, .T. ) ;
#15624=EDGE_CURVE ( 'NONE', #18734, #1692, #8900, .T. ) ;
#15636=CARTESIAN_POINT ( 'NONE',  ( 59.35000000000007248, 4.898587196589447341E-16, 3.999999999999378275 ) ) ;
#15654=DIRECTION ( 'NONE',  ( -1.000000000000000000, -0.000000000000000000, 1.047444401652940007E-14 ) ) ;
#15661=FACE_BOUND ( 'NONE', #1444, .T. ) ;
#15667=ORIENTED_EDGE ( 'NONE', *, *, #6290, .F. ) ;
#15675=VERTEX_POINT ( 'NONE', #13958 ) ;
#15679=ORIENTED_EDGE ( 'NONE', *, *, #27923, .T. ) ;
#15685=CARTESIAN_POINT ( 'NONE',  ( 68.05000000000002558, 1.401298464324817071E-42, -7.127859153248258291E-13 ) ) ;
#15714=DIRECTION ( 'NONE',  ( -1.000000000000000000, 0.000000000000000000, 1.047444401652940007E-14 ) ) ;
#15725=SHAPE_REPRESENTATION ( 'End Cap', ( #9018 ), #21749 ) ;
#15766=AXIS2_PLACEMENT_3D ( 'NONE', #15405, #3387, #3543 ) ;
#15778=ORIENTED_EDGE ( 'NONE', *, *, #15600, .T. ) ;
#15788=DIRECTION ( 'NONE',  ( 1.000000000000000000, -0.000000000000000000, -1.047444401652940007E-14 ) ) ;
#15823=CIRCLE ( 'NONE', #13272, 4.000000000000000000 ) ;
#15828=ORIENTED_EDGE ( 'NONE', *, *, #24625, .T. ) ;
#15853=ORIENTED_EDGE ( 'NONE', *, *, #3844, .F. ) ;
#15854=EDGE_CURVE ( 'NONE', #24915, #10286, #2873, .T. ) ;
#15855=CARTESIAN_POINT ( 'NONE',  ( 69.20000000000001705, 0.6441176470588244607, -1.707553061181374066 ) ) ;
#15913=CARTESIAN_POINT ( 'NONE',  ( 59.00000000000002132, 1.401298464324817071E-42, -6.179921969752347932E-13 ) ) ;
#15914=DIRECTION ( 'NONE',  ( -1.000000000000000000, 0.000000000000000000, 1.047444401652940007E-14 ) ) ;
#15943=AXIS2_PLACEMENT_3D ( 'NONE', #9071, #18746, #28386 ) ;
#15972=ADVANCED_FACE ( 'NONE', ( #24558 ), #13978, .F. ) ;
#15995=DIRECTION ( 'NONE',  ( -1.000000000000000000, 0.000000000000000000, 1.047444401652940007E-14 ) ) ;
#15998=DIRECTION ( 'NONE',  ( -1.000000000000000000, 0.000000000000000000, 1.047444401652940007E-14 ) ) ;
#16010=ADVANCED_FACE ( 'NONE', ( #28316 ), #13874, .T. ) ;
#16020=ORIENTED_EDGE ( 'NONE', *, *, #27958, .F. ) ;
#16032=AXIS2_PLACEMENT_3D ( 'NONE', #15913, #13540, #25421 ) ;
#16033=CIRCLE ( 'NONE', #21096, 0.2500000000000000000 ) ;
#16043=DIRECTION ( 'NONE',  ( 0.000000000000000000, 0.000000000000000000, 1.000000000000000000 ) ) ;
#16071=DIRECTION ( 'NONE',  ( 1.000000000000000000, 0.000000000000000000, -1.047444401652940007E-14 ) ) ;
#16157=COLOUR_RGB ( '', 0.72549020, 0.75294118, 0.79215686) ;
#16163=EDGE_CURVE ( 'NONE', #171, #1692, #19009, .T. ) ;
#16191=PRODUCT ( 'End Cap', 'End Cap', '', ( #22669 ) ) ;
#16205=DIRECTION ( 'NONE',  ( 0.000000000000000000, 0.000000000000000000, -1.000000000000000000 ) ) ;
#16232=ORIENTED_EDGE ( 'NONE', *, *, #16268, .T. ) ;
#16268=EDGE_CURVE ( 'NONE', #4097, #12947, #27070, .T. ) ;
#16284=CARTESIAN_POINT ( 'NONE',  ( 64.95000000000001705, 1.401298464324817071E-42, -6.803151388735846952E-13 ) ) ;
#16285=ORIENTED_EDGE ( 'NONE', *, *, #7232, .F. ) ;
#16294=AXIS2_PLACEMENT_3D ( 'NONE', #9629, #28922, #7235 ) ;
#16318=CARTESIAN_POINT ( 'NONE',  ( 68.95000000000003126, 1.401298464324817071E-42, -7.222129149397022450E-13 ) ) ;
#16324=LINE ( 'NONE', #1585, #19903 ) ;
#16325=AXIS2_PLACEMENT_3D ( 'NONE', #6241, #28247, #6557 ) ;
#16348=DIRECTION ( 'NONE',  ( 0.000000000000000000, 1.224646799147353947E-16, 1.000000000000000000 ) ) ;
#16352=CARTESIAN_POINT ( 'NONE',  ( 69.20000000000001705, -0.7500000000000000000, -2.238246715074081017 ) ) ;
#16367=TOROIDAL_SURFACE ( 'NONE', #14349, 0.3000000000000000444, 0.05000000000000000278 ) ;
#16368=CARTESIAN_POINT ( 'NONE',  ( 63.50000000000002842, 1.401298464324817071E-42, -6.651271950496169736E-13 ) ) ;
#16370=EDGE_LOOP ( 'NONE', ( #21579, #30825 ) ) ;
#16375=ADVANCED_FACE ( 'NONE', ( #5131 ), #19860, .F. ) ;
#16382=ORIENTED_EDGE ( 'NONE', *, *, #24625, .F. ) ;
#16398=ORIENTED_EDGE ( 'NONE', *, *, #15600, .F. ) ;
#16429=DIRECTION ( 'NONE',  ( 1.189524669241239105E-14, 0.000000000000000000, 1.000000000000000000 ) ) ;
#16437=EDGE_LOOP ( 'NONE', ( #24481, #30030 ) ) ;
#16450=ORIENTED_EDGE ( 'NONE', *, *, #7232, .T. ) ;
#16459=CIRCLE ( 'NONE', #2797, 4.000000000000000000 ) ;
#16482=FACE_OUTER_BOUND ( 'NONE', #28920, .T. ) ;
#16496=( NAMED_UNIT ( * ) PLANE_ANGLE_UNIT ( ) SI_UNIT ( $, .RADIAN. ) );
#16504=ORIENTED_EDGE ( 'NONE', *, *, #21109, .F. ) ;
#16561=FACE_OUTER_BOUND ( 'NONE', #16706, .T. ) ;
#16606=ADVANCED_FACE ( 'NONE', ( #2133 ), #26065, .T. ) ;
#16608=EDGE_CURVE ( 'NONE', #14417, #4801, #16459, .T. ) ;
#16652=CARTESIAN_POINT ( 'NONE',  ( 69.05000000000005400, 4.557543281186736018E-17, 3.020710678117922932 ) ) ;
#16666=DIRECTION ( 'NONE',  ( 0.000000000000000000, 0.000000000000000000, -1.000000000000000000 ) ) ;
#16672=DIRECTION ( 'NONE',  ( 9.188425696205898615E-15, 0.000000000000000000, 1.000000000000000000 ) ) ;
#16684=DIRECTION ( 'NONE',  ( 0.000000000000000000, -1.000000000000000000, -0.000000000000000000 ) ) ;
#16699=VERTEX_POINT ( 'NONE', #17477 ) ;
#16706=EDGE_LOOP ( 'NONE', ( #17641, #27490, #2343, #3094 ) ) ;
#16721=CARTESIAN_POINT ( 'NONE',  ( 59.35000000000002984, 1.401298464324817071E-42, -6.216582523810200043E-13 ) ) ;
#16723=CARTESIAN_POINT ( 'NONE',  ( 59.00000000000002132, 1.401298464324817071E-42, -6.179921969752347932E-13 ) ) ;
#16734=ORIENTED_EDGE ( 'NONE', *, *, #30775, .F. ) ;
#16749=VECTOR ( 'NONE', #5444, 1000.000000000000000 ) ;
#16791=FACE_BOUND ( 'NONE', #29474, .T. ) ;
#16829=EDGE_LOOP ( 'NONE', ( #10537, #15607, #13518, #29990 ) ) ;
#16842=EDGE_LOOP ( 'NONE', ( #8198, #17099, #13903, #5226 ) ) ;
#16844=CARTESIAN_POINT ( 'NONE',  ( 69.00000000000001421, 1.401298464324817071E-42, -7.227366371405287181E-13 ) ) ;
#16873=FILL_AREA_STYLE ('',( #14642 ) ) ;
#16879=AXIS2_PLACEMENT_3D ( 'NONE', #21441, #2256, #1775 ) ;
#16888=ORIENTED_EDGE ( 'NONE', *, *, #21365, .F. ) ;
#16909=DIRECTION ( 'NONE',  ( 1.000000000000000000, 0.000000000000000000, -1.047444401652940007E-14 ) ) ;
#16919=CIRCLE ( 'NONE', #3256, 1.875000000000000000 ) ;
#16956=ADVANCED_FACE ( 'NONE', ( #28533 ), #23562, .T. ) ;
#16960=LINE ( 'NONE', #17126, #25153 ) ;
#16982=FACE_OUTER_BOUND ( 'NONE', #24041, .T. ) ;
#16983=DIRECTION ( 'NONE',  ( 1.000000000000000000, -0.000000000000000000, -1.047444401652940007E-14 ) ) ;
#16996=ORIENTED_EDGE ( 'NONE', *, *, #670, .T. ) ;
#17010=ORIENTED_EDGE ( 'NONE', *, *, #31299, .T. ) ;
#17015=TOROIDAL_SURFACE ( 'NONE', #6873, 3.950000000000000178, 0.05000000000000000278 ) ;
#17029=CARTESIAN_POINT ( 'NONE',  ( 49.05000000000002558, 1.401298464324817071E-42, -5.137714790107672405E-13 ) ) ;
#17040=CARTESIAN_POINT ( 'NONE',  ( 68.00000000000004263, 1.401298464324817071E-42, 2.624999999999286793 ) ) ;
#17041=CIRCLE ( 'NONE', #21085, 3.500000000000000444 ) ;
#17074=AXIS2_PLACEMENT_3D ( 'NONE', #30866, #19002, #28811 ) ;
#17095=DIRECTION ( 'NONE',  ( 7.401486830834382195E-15, 0.000000000000000000, 1.000000000000000000 ) ) ;
#17099=ORIENTED_EDGE ( 'NONE', *, *, #27958, .T. ) ;
#17101=CYLINDRICAL_SURFACE ( 'NONE', #14285, 4.000000000000000000 ) ;
#17126=CARTESIAN_POINT ( 'NONE',  ( 69.25000000000004263, -0.5000000000000000000, 1.988246715072632620 ) ) ;
#17141=EDGE_CURVE ( 'NONE', #1976, #7542, #31144, .T. ) ;
#17169=PRODUCT_DEFINITION_FORMATION_WITH_SPECIFIED_SOURCE ( 'ANY', '', #16191, .NOT_KNOWN. ) ;
#17172=TOROIDAL_SURFACE ( 'NONE', #18195, 3.950000000000000178, 0.05000000000000000278 ) ;
#17186=DIRECTION ( 'NONE',  ( 1.282749433769087582E-30, 1.000000000000000000, 1.224646799147353207E-16 ) ) ;
#17235=ADVANCED_FACE ( 'NONE', ( #27082 ), #17015, .T. ) ;
#17238=EDGE_CURVE ( 'NONE', #26219, #20971, #2329, .T. ) ;
#17247=DIRECTION ( 'NONE',  ( -1.000000000000000000, 0.000000000000000000, 1.047444401652940007E-14 ) ) ;
#17267=ORIENTED_EDGE ( 'NONE', *, *, #20718, .T. ) ;
#17289=CIRCLE ( 'NONE', #15270, 0.2499999999999997780 ) ;
#17317=CARTESIAN_POINT ( 'NONE',  ( 63.50000000000000000, 0.8382352941176473005, -2.222158093317947003 ) ) ;
#17321=CARTESIAN_POINT ( 'NONE',  ( 68.00000000000000000, 0.6617647058823536987, -1.754335336830146641 ) ) ;
#17328=EDGE_CURVE ( 'NONE', #10580, #6314, #9412, .T. ) ;
#17338=AXIS2_PLACEMENT_3D ( 'NONE', #16368, #22882, #18605 ) ;
#17377=DIRECTION ( 'NONE',  ( -1.047444401652940007E-14, 0.000000000000000000, -1.000000000000000000 ) ) ;
#17406=CARTESIAN_POINT ( 'NONE',  ( 69.20000000000003126, 1.401298464324817071E-42, -7.248315259438346108E-13 ) ) ;
#17417=CARTESIAN_POINT ( 'NONE',  ( 68.00000000000004263, 0.5000000000000000000, 1.988246715072644166 ) ) ;
#17443=CARTESIAN_POINT ( 'NONE',  ( 69.01464466094067518, 4.111760188415125337E-16, -2.985355339060038027 ) ) ;
#17476=CARTESIAN_POINT ( 'NONE',  ( 64.95000000000005969, 4.898587196589412829E-16, 3.999999999999320099 ) ) ;
#17477=CARTESIAN_POINT ( 'NONE',  ( 69.20000000000005969, 0.8382352941176473005, 2.222158093316557004 ) ) ;
#17501=EDGE_LOOP ( 'NONE', ( #19989, #21275, #326, #22558 ) ) ;
#17537=EDGE_CURVE ( 'NONE', #23786, #10712, #23912, .T. ) ;
#17542=DIRECTION ( 'NONE',  ( 1.000000000000000000, 0.000000000000000000, -1.047444401652940007E-14 ) ) ;
#17554=AXIS2_PLACEMENT_3D ( 'NONE', #17915, #808, #17767 ) ;
#17555=EDGE_CURVE ( 'NONE', #31290, #29622, #6820, .T. ) ;
#17557=AXIS2_PLACEMENT_3D ( 'NONE', #16723, #3506, #27723 ) ;
#17568=ADVANCED_FACE ( 'NONE', ( #18308 ), #19977, .T. ) ;
#17584=ORIENTED_EDGE ( 'NONE', *, *, #12959, .T. ) ;
#17619=CARTESIAN_POINT ( 'NONE',  ( 69.20000000000003126, 4.557543281186736018E-17, -7.248315259438346108E-13 ) ) ;
#17641=ORIENTED_EDGE ( 'NONE', *, *, #4142, .F. ) ;
#17654=DIRECTION ( 'NONE',  ( 1.000000000000000000, 0.000000000000000000, -1.047444401652940007E-14 ) ) ;
#17660=AXIS2_PLACEMENT_3D ( 'NONE', #28070, #22877, #8293 ) ;
#17688=CARTESIAN_POINT ( 'NONE',  ( 60.67929986713514978, 1.401298464324817071E-42, -6.355819294205068152E-13 ) ) ;
#17763=CARTESIAN_POINT ( 'NONE',  ( 49.00000000000000000, -0.7500000000000000000, -1.988246715073871185 ) ) ;
#17767=DIRECTION ( 'NONE',  ( 9.297243531610763781E-15, 0.000000000000000000, 1.000000000000000000 ) ) ;
#17774=CARTESIAN_POINT ( 'NONE',  ( 69.20000000000004547, 0.4500000000000000111, 1.988246715072634396 ) ) ;
#17782=EDGE_CURVE ( 'NONE', #28026, #6108, #19472, .T. ) ;
#17805=DIRECTION ( 'NONE',  ( 1.000000000000000000, 0.000000000000000000, -1.047444401652940007E-14 ) ) ;
#17901=EDGE_CURVE ( 'NONE', #2745, #3817, #20981, .T. ) ;
#17906=AXIS2_PLACEMENT_3D ( 'NONE', #26776, #26304, #23932 ) ;
#17915=CARTESIAN_POINT ( 'NONE',  ( 69.01464466094070360, 4.557543281186736018E-17, -7.228900318216929560E-13 ) ) ;
#17928=AXIS2_PLACEMENT_3D ( 'NONE', #3295, #25139, #27205 ) ;
#17949=CARTESIAN_POINT ( 'NONE',  ( 68.05000000000006821, 1.401298464324817071E-42, 3.949999999999287414 ) ) ;
#17960=TOROIDAL_SURFACE ( 'NONE', #29558, 0.3000000000000000444, 0.05000000000000000278 ) ;
#17989=CARTESIAN_POINT ( 'NONE',  ( 49.00000000000000000, 0.6617647058823536987, -1.754335336829947467 ) ) ;
#18014=CARTESIAN_POINT ( 'NONE',  ( 63.50000000000000000, 1.401298464324817071E-42, -2.375000000000663913 ) ) ;
#18027=CIRCLE ( 'NONE', #6392, 0.2500000000000000000 ) ;
#18050=TOROIDAL_SURFACE ( 'NONE', #4386, 0.3000000000000000444, 0.05000000000000000278 ) ;
#18104=ORIENTED_EDGE ( 'NONE', *, *, #1422, .F. ) ;
#18119=CYLINDRICAL_SURFACE ( 'NONE', #30160, 2.874999999999999112 ) ;
#18124=AXIS2_PLACEMENT_3D ( 'NONE', #29728, #29556, #25132 ) ;
#18172=EDGE_LOOP ( 'NONE', ( #26713, #12758, #5937, #24986, #17584, #474, #16232 ) ) ;
#18178=EDGE_CURVE ( 'NONE', #3064, #21345, #8836, .T. ) ;
#18195=AXIS2_PLACEMENT_3D ( 'NONE', #6055, #30557, #13456 ) ;
#18210=ORIENTED_EDGE ( 'NONE', *, *, #10374, .F. ) ;
#18273=DIRECTION ( 'NONE',  ( 1.000000000000000000, -0.000000000000000000, -1.047444401652940007E-14 ) ) ;
#18286=CYLINDRICAL_SURFACE ( 'NONE', #17338, 2.374999999999998668 ) ;
#18308=FACE_OUTER_BOUND ( 'NONE', #7325, .T. ) ;
#18309=TOROIDAL_SURFACE ( 'NONE', #21980, 1.824999999999998623, 0.05000000000000000278 ) ;
#18316=ORIENTED_EDGE ( 'NONE', *, *, #7209, .F. ) ;
#18337=ORIENTED_EDGE ( 'NONE', *, *, #17141, .F. ) ;
#18359=CARTESIAN_POINT ( 'NONE',  ( 68.00000000000004263, 0.7500000000000000000, 1.988246715072644166 ) ) ;
#18360=EDGE_LOOP ( 'NONE', ( #14151, #28213, #11783, #8692 ) ) ;
#18368=AXIS2_PLACEMENT_3D ( 'NONE', #19384, #6866, #24130 ) ;
#18384=AXIS2_PLACEMENT_3D ( 'NONE', #30370, #8673, #6306 ) ;
#18457=EDGE_CURVE ( 'NONE', #865, #31227, #25569, .T. ) ;
#18531=AXIS2_PLACEMENT_3D ( 'NONE', #24521, #9977, #2689 ) ;
#18573=VECTOR ( 'NONE', #7141, 1000.000000000000000 ) ;
#18605=DIRECTION ( 'NONE',  ( -1.168655815394902336E-14, 0.000000000000000000, -1.000000000000000000 ) ) ;
#18609=FACE_OUTER_BOUND ( 'NONE', #3526, .T. ) ;
#18689=ADVANCED_FACE ( 'NONE', ( #29900, #15661 ), #13254, .T. ) ;
#18734=VERTEX_POINT ( 'NONE', #27370 ) ;
#18737=AXIS2_PLACEMENT_3D ( 'NONE', #29997, #16071, #25724 ) ;
#18746=DIRECTION ( 'NONE',  ( 1.000000000000000000, 0.000000000000000000, -1.047444401652940007E-14 ) ) ;
#18768=CARTESIAN_POINT ( 'NONE',  ( 69.00000000000005684, 4.557543281186736018E-17, 3.020710678117923376 ) ) ;
#18787=CARTESIAN_POINT ( 'NONE',  ( 63.50000000000005684, 2.908536147974998226E-16, 2.374999999999333422 ) ) ;
#18804=ORIENTED_EDGE ( 'NONE', *, *, #5935, .F. ) ;
#18813=CIRCLE ( 'NONE', #15766, 0.04999999999999449329 ) ;
#18817=EDGE_CURVE ( 'NONE', #27508, #1976, #3317, .T. ) ;
#18845=DIRECTION ( 'NONE',  ( 1.000000000000000000, 0.000000000000000000, -1.047444401652940007E-14 ) ) ;
#18863=FACE_BOUND ( 'NONE', #22105, .T. ) ;
#18865=EDGE_CURVE ( 'NONE', #23750, #27662, #2328, .T. ) ;
#18891=DIRECTION ( 'NONE',  ( -1.047444401652940007E-14, 0.000000000000000000, -1.000000000000000000 ) ) ;
#18898=CARTESIAN_POINT ( 'NONE',  ( 49.00000000000000000, 0.7500000000000000000, -1.988246715073871629 ) ) ;
#18929=EDGE_CURVE ( 'NONE', #13465, #21838, #24482, .T. ) ;
#18933=DIRECTION ( 'NONE',  ( 1.000000000000000000, 0.000000000000000000, -1.047444401652940007E-14 ) ) ;
#18935=ORIENTED_EDGE ( 'NONE', *, *, #8165, .T. ) ;
#18936=EDGE_CURVE ( 'NONE', #13707, #27904, #15452, .T. ) ;
#18941=AXIS2_PLACEMENT_3D ( 'NONE', #25942, #25470, #21225 ) ;
#18945=AXIS2_PLACEMENT_3D ( 'NONE', #25641, #2911, #10185 ) ;
#18946=EDGE_LOOP ( 'NONE', ( #30208, #30478, #31, #28576 ) ) ;
#18972=EDGE_CURVE ( 'NONE', #15234, #25083, #12291, .T. ) ;
#18986=AXIS2_PLACEMENT_3D ( 'NONE', #13163, #15714, #25360 ) ;
#19002=DIRECTION ( 'NONE',  ( 1.000000000000000000, -0.000000000000000000, -1.047444401652940007E-14 ) ) ;
#19009=CIRCLE ( 'NONE', #7857, 0.2499999999999997780 ) ;
#19011=PLANE ( 'NONE',  #3869 ) ;
#19020=DIRECTION ( 'NONE',  ( 1.047444401652940007E-14, 0.000000000000000000, 1.000000000000000000 ) ) ;
#19135=CIRCLE ( 'NONE', #30221, 0.2500000000000000000 ) ;
#19144=EDGE_CURVE ( 'NONE', #3817, #13707, #5362, .T. ) ;
#19171=FACE_OUTER_BOUND ( 'NONE', #14453, .T. ) ;
#19184=EDGE_CURVE ( 'NONE', #16699, #24542, #5646, .T. ) ;
#19217=DIRECTION ( 'NONE',  ( 0.000000000000000000, -3.469446951953611033E-15, 1.000000000000000000 ) ) ;
#19234=CYLINDRICAL_SURFACE ( 'NONE', #31134, 3.500000000000000444 ) ;
#19235=AXIS2_PLACEMENT_3D ( 'NONE', #11369, #11848, #28799 ) ;
#19250=FACE_OUTER_BOUND ( 'NONE', #6522, .T. ) ;
#19266=FACE_BOUND ( 'NONE', #27527, .T. ) ;
#19276=CARTESIAN_POINT ( 'NONE',  ( 68.00000000000001421, 1.401298464324817071E-42, -7.122621931239992550E-13 ) ) ;
#19291=DIRECTION ( 'NONE',  ( 1.057355261547768637E-14, 0.000000000000000000, 1.000000000000000000 ) ) ;
#19312=LINE ( 'NONE', #10253, #1385 ) ;
#19336=AXIS2_PLACEMENT_3D ( 'NONE', #6796, #23589, #6641 ) ;
#19355=EDGE_CURVE ( 'NONE', #4097, #16699, #305, .T. ) ;
#19358=SURFACE_STYLE_USAGE ( .BOTH. , #23792 ) ;
#19384=CARTESIAN_POINT ( 'NONE',  ( 49.00000000000002132, 3.252606517456513302E-16, -5.132477568099407673E-13 ) ) ;
#19427=EDGE_LOOP ( 'NONE', ( #430, #26964, #3789, #6212 ) ) ;
#19431=DIRECTION ( 'NONE',  ( 0.000000000000000000, -8.673617379884043361E-16, 1.000000000000000000 ) ) ;
#19449=AXIS2_PLACEMENT_3D ( 'NONE', #9961, #17247, #19635 ) ;
#19472=CIRCLE ( 'NONE', #4778, 3.000000000000000000 ) ;
#19494=DIRECTION ( 'NONE',  ( -1.000000000000000000, -0.000000000000000000, 1.047444401652940007E-14 ) ) ;
#19499=EDGE_CURVE ( 'NONE', #30383, #23530, #6927, .T. ) ;
#19500=DIRECTION ( 'NONE',  ( -1.000000000000000000, -0.000000000000000000, 1.047444401652940007E-14 ) ) ;
#19528=CARTESIAN_POINT ( 'NONE',  ( 69.20000000000005969, 0.8558823529411765385, 2.268940368965341126 ) ) ;
#19553=AXIS2_PLACEMENT_3D ( 'NONE', #5138, #14938, #7362 ) ;
#19565=CARTESIAN_POINT ( 'NONE',  ( 49.04999999999999716, 3.275930187719168862E-16, -2.675000000000512745 ) ) ;
#19588=ORIENTED_EDGE ( 'NONE', *, *, #28566, .T. ) ;
#19590=CARTESIAN_POINT ( 'NONE',  ( 68.00000000000000000, 0.7500000000000000000, -1.988246715074070581 ) ) ;
#19606=CIRCLE ( 'NONE', #25631, 4.000000000000000000 ) ;
#19612=CARTESIAN_POINT ( 'NONE',  ( 63.50000000000005684, 2.908536147974962234E-16, 2.374999999999333422 ) ) ;
#19623=FACE_OUTER_BOUND ( 'NONE', #11463, .T. ) ;
#19625=ORIENTED_EDGE ( 'NONE', *, *, #26310, .F. ) ;
#19635=DIRECTION ( 'NONE',  ( 1.057355261547768637E-14, 0.000000000000000000, 1.000000000000000000 ) ) ;
#19653=ORIENTED_EDGE ( 'NONE', *, *, #30535, .F. ) ;
#19669=DIRECTION ( 'NONE',  ( -1.000000000000000000, -0.000000000000000000, 1.047444401652940007E-14 ) ) ;
#19671=ADVANCED_FACE ( 'NONE', ( #28831, #18863 ), #11727, .F. ) ;
#19677=CARTESIAN_POINT ( 'NONE',  ( 69.20000000000003126, 3.252606517456513302E-16, -7.248315259438346108E-13 ) ) ;
#19731=AXIS2_PLACEMENT_3D ( 'NONE', #23604, #4263, #27721 ) ;
#19748=ORIENTED_EDGE ( 'NONE', *, *, #9078, .T. ) ;
#19773=CARTESIAN_POINT ( 'NONE',  ( 69.20000000000001705, 0.7500000000000000000, -1.988246715074083237 ) ) ;
#19775=DIRECTION ( 'NONE',  ( 0.000000000000000000, 0.000000000000000000, -1.000000000000000000 ) ) ;
#19790=EDGE_CURVE ( 'NONE', #24431, #4809, #28618, .T. ) ;
#19814=ADVANCED_FACE ( 'NONE', ( #23725 ), #30986, .T. ) ;
#19823=CIRCLE ( 'NONE', #30424, 2.674999999999998934 ) ;
#19831=DIRECTION ( 'NONE',  ( 1.009293658750142281E-14, 0.000000000000000000, 1.000000000000000000 ) ) ;
#19836=CYLINDRICAL_SURFACE ( 'NONE', #13969, 0.2500000000000002220 ) ;
#19849=ADVANCED_FACE ( 'NONE', ( #26397 ), #14519, .F. ) ;
#19853=EDGE_LOOP ( 'NONE', ( #1673, #25899, #28436, #16888 ) ) ;
#19860=CYLINDRICAL_SURFACE ( 'NONE', #14441, 0.2500000000000000000 ) ;
#19865=EDGE_CURVE ( 'NONE', #21345, #3064, #28666, .T. ) ;
#19867=DIRECTION ( 'NONE',  ( -1.000000000000000000, 0.000000000000000000, 1.047444401652940007E-14 ) ) ;
#19869=LINE ( 'NONE', #17040, #1322 ) ;
#19894=ORIENTED_EDGE ( 'NONE', *, *, #6848, .F. ) ;
#19903=VECTOR ( 'NONE', #6814, 1000.000000000000000 ) ;
#19914=ORIENTED_EDGE ( 'NONE', *, *, #11732, .T. ) ;
#19941=CIRCLE ( 'NONE', #18941, 2.624999999999998668 ) ;
#19946=ORIENTED_EDGE ( 'NONE', *, *, #21694, .T. ) ;
#19977=TOROIDAL_SURFACE ( 'NONE', #3270, 3.950000000000000178, 0.05000000000000000278 ) ;
#19982=EDGE_CURVE ( 'NONE', #24785, #30539, #7994, .T. ) ;
#19985=DIRECTION ( 'NONE',  ( 3.696862594069216125E-15, 0.9356455129756975353, 0.3529411764705897570 ) ) ;
#19986=DIRECTION ( 'NONE',  ( 0.000000000000000000, 0.000000000000000000, -1.000000000000000000 ) ) ;
#19989=ORIENTED_EDGE ( 'NONE', *, *, #10190, .F. ) ;
#20079=ORIENTED_EDGE ( 'NONE', *, *, #27093, .F. ) ;
#20092=CIRCLE ( 'NONE', #12988, 0.05000000000000012768 ) ;
#20102=DIRECTION ( 'NONE',  ( 1.057355261547768637E-14, 0.000000000000000000, 1.000000000000000000 ) ) ;
#20103=AXIS2_PLACEMENT_3D ( 'NONE', #19565, #17186, #26830 ) ;
#20168=ORIENTED_EDGE ( 'NONE', *, *, #460, .T. ) ;
#20240=CARTESIAN_POINT ( 'NONE',  ( 69.25000000000004263, 0.6441176470588245717, 1.707553061179924114 ) ) ;
#20250=CIRCLE ( 'NONE', #24281, 2.374999999999998668 ) ;
#20260=CIRCLE ( 'NONE', #28330, 3.950000000000000178 ) ;
#20267=EDGE_LOOP ( 'NONE', ( #24487, #19748, #28732, #24036 ) ) ;
#20277=DIRECTION ( 'NONE',  ( 0.000000000000000000, -0.3529411764705863708, 0.9356455129756987565 ) ) ;
#20286=DIRECTION ( 'NONE',  ( 1.000000000000000000, 0.000000000000000000, -1.047444401652940007E-14 ) ) ;
#20293=SHAPE_DEFINITION_REPRESENTATION ( #6837, #15725 ) ;
#20314=DIRECTION ( 'NONE',  ( 9.824982518806699669E-15, 0.000000000000000000, 1.000000000000000000 ) ) ;
#20335=CARTESIAN_POINT ( 'NONE',  ( 69.20000000000001705, -0.4500000000000000111, -1.988246715074081017 ) ) ;
#20362=EDGE_CURVE ( 'NONE', #27904, #13707, #8355, .T. ) ;
#20380=DIRECTION ( 'NONE',  ( 0.000000000000000000, 1.224646799147353207E-16, 1.000000000000000000 ) ) ;
#20413=AXIS2_PLACEMENT_3D ( 'NONE', #17406, #27052, #5368 ) ;
#20415=AXIS2_PLACEMENT_3D ( 'NONE', #12536, #19985, #29179 ) ;
#20474=ORIENTED_EDGE ( 'NONE', *, *, #16268, .F. ) ;
#20509=ORIENTED_EDGE ( 'NONE', *, *, #16163, .F. ) ;
#20539=DIRECTION ( 'NONE',  ( 0.000000000000000000, 0.000000000000000000, -1.000000000000000000 ) ) ;
#20581=AXIS2_PLACEMENT_3D ( 'NONE', #20624, #15998, #6049 ) ;
#20600=CIRCLE ( 'NONE', #24109, 0.05000000000000012768 ) ;
#20603=AXIS2_PLACEMENT_3D ( 'NONE', #15448, #25099, #20380 ) ;
#20623=CARTESIAN_POINT ( 'NONE',  ( 69.20000000000001705, -0.7500000000000000000, -1.988246715074081017 ) ) ;
#20624=CARTESIAN_POINT ( 'NONE',  ( 69.23535533905935324, 4.557543281186736018E-17, -7.252018534634969470E-13 ) ) ;
#20640=DIRECTION ( 'NONE',  ( 0.000000000000000000, -0.3529411764705844834, 0.9356455129756994227 ) ) ;
#20649=EDGE_LOOP ( 'NONE', ( #6016, #14094, #18210, #23211 ) ) ;
#20670=DIRECTION ( 'NONE',  ( 1.047444401652940007E-14, 0.000000000000000000, 1.000000000000000000 ) ) ;
#20684=ORIENTED_EDGE ( 'NONE', *, *, #24446, .F. ) ;
#20691=EDGE_CURVE ( 'NONE', #2745, #27904, #2696, .T. ) ;
#20700=DIRECTION ( 'NONE',  ( 1.000000000000000000, 0.000000000000000000, -1.047444401652940007E-14 ) ) ;
#20718=EDGE_CURVE ( 'NONE', #12947, #21492, #11285, .T. ) ;
#20739=VERTEX_POINT ( 'NONE', #12645 ) ;
#20742=CYLINDRICAL_SURFACE ( 'NONE', #18384, 0.2500000000000002220 ) ;
#20759=FACE_OUTER_BOUND ( 'NONE', #19853, .T. ) ;
#20806=CARTESIAN_POINT ( 'NONE',  ( 68.94999999999998863, 1.401298464324817071E-42, -4.000000000000722977 ) ) ;
#20819=ADVANCED_FACE ( 'NONE', ( #617 ), #14817, .T. ) ;
#20826=DIRECTION ( 'NONE',  ( -1.000000000000000000, -0.000000000000000000, 1.047444401652940007E-14 ) ) ;
#20833=CARTESIAN_POINT ( 'NONE',  ( 49.04999999999999716, 3.214697847761800597E-16, -2.625000000000512923 ) ) ;
#20834=DIRECTION ( 'NONE',  ( 0.000000000000000000, 0.000000000000000000, -1.000000000000000000 ) ) ;
#20864=CARTESIAN_POINT ( 'NONE',  ( 67.99999999999998579, 4.867971026610729436E-16, -3.950000000000712497 ) ) ;
#20881=ADVANCED_FACE ( 'NONE', ( #11062 ), #20742, .F. ) ;
#20918=AXIS2_PLACEMENT_3D ( 'NONE', #16844, #28871, #13798 ) ;
#20954=DIRECTION ( 'NONE',  ( 1.000000000000000000, -0.000000000000000000, -1.047444401652940007E-14 ) ) ;
#20960=TOROIDAL_SURFACE ( 'NONE', #6779, 2.729289321881338548, 0.05000000000000000278 ) ;
#20962=VERTEX_POINT ( 'NONE', #6776 ) ;
#20969=FACE_BOUND ( 'NONE', #21281, .T. ) ;
#20971=VERTEX_POINT ( 'NONE', #11844 ) ;
#20981=CIRCLE ( 'NONE', #23502, 2.874999999999999112 ) ;
#20997=EDGE_CURVE ( 'NONE', #8754, #5843, #29986, .T. ) ;
#20999=DIRECTION ( 'NONE',  ( 0.000000000000000000, 0.000000000000000000, -1.000000000000000000 ) ) ;
#21014=VERTEX_POINT ( 'NONE', #20240 ) ;
#21017=ORIENTED_EDGE ( 'NONE', *, *, #24226, .T. ) ;
#21022=AXIS2_PLACEMENT_3D ( 'NONE', #29596, #19500, #24395 ) ;
#21044=DIRECTION ( 'NONE',  ( -1.000000000000000000, 0.000000000000000000, 1.047444401652940007E-14 ) ) ;
#21048=CARTESIAN_POINT ( 'NONE',  ( 59.00000000000005684, 1.401298464324817071E-42, 2.999999999999382272 ) ) ;
#21081=ADVANCED_FACE ( 'NONE', ( #29543 ), #16367, .T. ) ;
#21082=AXIS2_PLACEMENT_3D ( 'NONE', #6935, #7092, #19291 ) ;
#21085=AXIS2_PLACEMENT_3D ( 'NONE', #7283, #14400, #24380 ) ;
#21088=AXIS2_PLACEMENT_3D ( 'NONE', #1869, #11539, #30845 ) ;
#21091=CARTESIAN_POINT ( 'NONE',  ( 49.00000000000004974, 3.520859547548639454E-16, 2.874999999999486189 ) ) ;
#21096=AXIS2_PLACEMENT_3D ( 'NONE', #8133, #17805, #537 ) ;
#21100=DIRECTION ( 'NONE',  ( -1.047444401652940007E-14, 0.000000000000000000, -1.000000000000000000 ) ) ;
#21109=EDGE_CURVE ( 'NONE', #4801, #14417, #7766, .T. ) ;
#21118=ORIENTED_EDGE ( 'NONE', *, *, #859, .T. ) ;
#21142=AXIS2_PLACEMENT_3D ( 'NONE', #4686, #21668, #9623 ) ;
#21143=ORIENTED_EDGE ( 'NONE', *, *, #19790, .F. ) ;
#21147=ORIENTED_EDGE ( 'NONE', *, *, #25539, .F. ) ;
#21165=DIRECTION ( 'NONE',  ( 0.000000000000000000, 0.000000000000000000, -1.000000000000000000 ) ) ;
#21218=ORIENTED_EDGE ( 'NONE', *, *, #21109, .T. ) ;
#21225=DIRECTION ( 'NONE',  ( 1.057355261547768637E-14, 0.000000000000000000, 1.000000000000000000 ) ) ;
#21242=DIRECTION ( 'NONE',  ( -1.047444401652940007E-14, 0.000000000000000000, -1.000000000000000000 ) ) ;
#21275=ORIENTED_EDGE ( 'NONE', *, *, #16608, .F. ) ;
#21281=EDGE_LOOP ( 'NONE', ( #13459, #7309 ) ) ;
#21328=DIRECTION ( 'NONE',  ( -7.604267291953127011E-15, 0.000000000000000000, -1.000000000000000000 ) ) ;
#21345=VERTEX_POINT ( 'NONE', #22991 ) ;
#21353=ORIENTED_EDGE ( 'NONE', *, *, #21690, .T. ) ;
#21365=EDGE_CURVE ( 'NONE', #6138, #4566, #23970, .T. ) ;
#21378=ORIENTED_EDGE ( 'NONE', *, *, #30738, .F. ) ;
#21395=CARTESIAN_POINT ( 'NONE',  ( 48.99999999999999289, 3.490243377569955075E-16, -2.825000000000512212 ) ) ;
#21410=CARTESIAN_POINT ( 'NONE',  ( 69.20000000000004547, -0.7500000000000000000, 1.988246715072631732 ) ) ;
#21414=EDGE_CURVE ( 'NONE', #5901, #15234, #2716, .T. ) ;
#21441=CARTESIAN_POINT ( 'NONE',  ( 69.20000000000001705, -0.7500000000000000000, -1.988246715074081017 ) ) ;
#21446=CARTESIAN_POINT ( 'NONE',  ( 59.35000000000002984, 1.401298464324817071E-42, -6.216582523810200043E-13 ) ) ;
#21468=FACE_OUTER_BOUND ( 'NONE', #20649, .T. ) ;
#21486=CARTESIAN_POINT ( 'NONE',  ( 63.50000000000000000, 0.7500000000000000000, -1.988246715074021731 ) ) ;
#21492=VERTEX_POINT ( 'NONE', #28687 ) ;
#21507=CARTESIAN_POINT ( 'NONE',  ( 49.00000000000000000, -0.5000000000000000000, -1.988246715073869408 ) ) ;
#21513=DIRECTION ( 'NONE',  ( 1.000000000000000000, -0.000000000000000000, -1.047444401652940007E-14 ) ) ;
#21515=ORIENTED_EDGE ( 'NONE', *, *, #14511, .T. ) ;
#21520=DIRECTION ( 'NONE',  ( -1.000000000000000000, 0.000000000000000000, 1.047444401652940007E-14 ) ) ;
#21521=ORIENTED_EDGE ( 'NONE', *, *, #8089, .T. ) ;
#21551=DIRECTION ( 'NONE',  ( 1.000000000000000000, -0.000000000000000000, -1.047444401652940007E-14 ) ) ;
#21561=ORIENTED_EDGE ( 'NONE', *, *, #17901, .T. ) ;
#21574=CIRCLE ( 'NONE', #29625, 0.04999999999999994033 ) ;
#21579=ORIENTED_EDGE ( 'NONE', *, *, #738, .T. ) ;
#21582=VECTOR ( 'NONE', #5903, 1000.000000000000000 ) ;
#21586=ORIENTED_EDGE ( 'NONE', *, *, #20718, .F. ) ;
#21591=CARTESIAN_POINT ( 'NONE',  ( 68.95000000000003126, 1.401298464324817071E-42, -7.222129149397022450E-13 ) ) ;
#21598=DIRECTION ( 'NONE',  ( 1.040834085586084257E-14, 0.000000000000000000, 1.000000000000000000 ) ) ;
#21613=AXIS2_PLACEMENT_3D ( 'NONE', #5218, #15035, #15341 ) ;
#21663=ORIENTED_EDGE ( 'NONE', *, *, #17238, .T. ) ;
#21668=DIRECTION ( 'NONE',  ( -1.000000000000000000, -0.000000000000000000, 1.047444401652940007E-14 ) ) ;
#21670=ORIENTED_EDGE ( 'NONE', *, *, #30738, .T. ) ;
#21671=CARTESIAN_POINT ( 'NONE',  ( 59.35000000000006537, 1.401298464324817071E-42, 3.499999999999379163 ) ) ;
#21679=DIRECTION ( 'NONE',  ( 9.912705577010325352E-15, 0.000000000000000000, 1.000000000000000000 ) ) ;
#21690=EDGE_CURVE ( 'NONE', #18734, #20962, #30031, .T. ) ;
#21693=EDGE_LOOP ( 'NONE', ( #31116, #12540, #16285, #4659 ) ) ;
#21694=EDGE_CURVE ( 'NONE', #10712, #8546, #16919, .T. ) ;
#21705=CARTESIAN_POINT ( 'NONE',  ( 48.99999999999999289, 3.275930187719168862E-16, -2.675000000000511857 ) ) ;
#21707=DIRECTION ( 'NONE',  ( 1.000000000000000000, 0.000000000000000000, -1.047444401652940007E-14 ) ) ;
#21743=ADVANCED_FACE ( 'NONE', ( #26 ), #20960, .T. ) ;
#21749=( GEOMETRIC_REPRESENTATION_CONTEXT ( 3 ) GLOBAL_UNCERTAINTY_ASSIGNED_CONTEXT ( ( #6017 ) ) GLOBAL_UNIT_ASSIGNED_CONTEXT ( ( #6831, #16496, #26153 ) ) REPRESENTATION_CONTEXT ( 'NONE', 'WORKASPACE' ) );
#21780=VERTEX_POINT ( 'NONE', #1102 ) ;
#21801=DIRECTION ( 'NONE',  ( 0.000000000000000000, 0.000000000000000000, -1.000000000000000000 ) ) ;
#21838=VERTEX_POINT ( 'NONE', #17417 ) ;
#21861=CIRCLE ( 'NONE', #12709, 0.2999999999999999334 ) ;
#21883=ORIENTED_EDGE ( 'NONE', *, *, #29823, .T. ) ;
#21902=EDGE_CURVE ( 'NONE', #8529, #6314, #19941, .T. ) ;
#21924=ORIENTED_EDGE ( 'NONE', *, *, #28945, .T. ) ;
#21925=CARTESIAN_POINT ( 'NONE',  ( 68.05000000000002558, 1.401298464324817071E-42, -7.127859153248258291E-13 ) ) ;
#21933=CARTESIAN_POINT ( 'NONE',  ( 69.20000000000001705, -0.7500000000000000000, -1.988246715074081017 ) ) ;
#21934=AXIS2_PLACEMENT_3D ( 'NONE', #24690, #12795, #8217 ) ;
#21972=DIRECTION ( 'NONE',  ( 1.037591611799212092E-14, 0.000000000000000000, 1.000000000000000000 ) ) ;
#21980=AXIS2_PLACEMENT_3D ( 'NONE', #5051, #21707, #8091 ) ;
#22028=EDGE_LOOP ( 'NONE', ( #4919, #22453, #27191, #9627 ) ) ;
#22036=ORIENTED_EDGE ( 'NONE', *, *, #12527, .T. ) ;
#22044=FACE_BOUND ( 'NONE', #18172, .T. ) ;
#22049=AXIS2_PLACEMENT_3D ( 'NONE', #15060, #16983, #19217 ) ;
#22097=DIRECTION ( 'NONE',  ( 0.000000000000000000, -0.3529411764705897014, -0.9356455129756974243 ) ) ;
#22105=EDGE_LOOP ( 'NONE', ( #21017, #15828 ) ) ;
#22115=CARTESIAN_POINT ( 'NONE',  ( 69.20000000000005969, -0.8382352941176473005, 2.222158093316557004 ) ) ;
#22132=AXIS2_PLACEMENT_3D ( 'NONE', #14602, #24267, #25015 ) ;
#22147=VECTOR ( 'NONE', #7395, 1000.000000000000000 ) ;
#22155=CIRCLE ( 'NONE', #14034, 2.874999999999999112 ) ;
#22285=CIRCLE ( 'NONE', #18737, 1.824999999999998623 ) ;
#22287=DIRECTION ( 'NONE',  ( 1.000000000000000000, 0.000000000000000000, -1.047444401652940007E-14 ) ) ;
#22300=EDGE_LOOP ( 'NONE', ( #7180, #10750, #17267, #30521 ) ) ;
#22329=ADVANCED_FACE ( 'NONE', ( #5990 ), #26005, .T. ) ;
#22343=CARTESIAN_POINT ( 'NONE',  ( 68.00000000000000000, -0.5000000000000000000, -1.988246715074070137 ) ) ;
#22353=DIRECTION ( 'NONE',  ( -1.047444401652940007E-14, 0.000000000000000000, -1.000000000000000000 ) ) ;
#22355=CARTESIAN_POINT ( 'NONE',  ( 69.25000000000001421, 3.252606517456513302E-16, -7.253552481446610839E-13 ) ) ;
#22375=EDGE_LOOP ( 'NONE', ( #9969, #6451, #30689, #9540 ) ) ;
#22415=ORIENTED_EDGE ( 'NONE', *, *, #28566, .F. ) ;
#22453=ORIENTED_EDGE ( 'NONE', *, *, #27708, .T. ) ;
#22454=CARTESIAN_POINT ( 'NONE',  ( 64.94999999999997442, 1.401298464324817071E-42, -3.950000000000680522 ) ) ;
#22493=DIRECTION ( 'NONE',  ( 1.168655815394902336E-14, 0.000000000000000000, 1.000000000000000000 ) ) ;
#22509=DIRECTION ( 'NONE',  ( -1.000000000000000000, 0.000000000000000000, 1.047444401652940007E-14 ) ) ;
#22522=ADVANCED_FACE ( 'NONE', ( #7226 ), #23508, .T. ) ;
#22538=VECTOR ( 'NONE', #7701, 1000.000000000000000 ) ;
#22558=ORIENTED_EDGE ( 'NONE', *, *, #18817, .T. ) ;
#22571=EDGE_CURVE ( 'NONE', #8746, #9260, #30044, .T. ) ;
#22586=DIRECTION ( 'NONE',  ( -0.7071067811865413555, 0.000000000000000000, 0.7071067811865536790 ) ) ;
#22609=CARTESIAN_POINT ( 'NONE',  ( 69.20000000000001705, 0.7500000000000000000, -1.988246715074081017 ) ) ;
#22621=CIRCLE ( 'NONE', #30190, 3.500000000000000444 ) ;
#22655=VECTOR ( 'NONE', #26517, 1000.000000000000000 ) ;
#22661=ORIENTED_EDGE ( 'NONE', *, *, #9899, .T. ) ;
#22669=PRODUCT_CONTEXT ( 'NONE', #12352, 'mechanical' ) ;
#22670=CIRCLE ( 'NONE', #7487, 2.874999999999999112 ) ;
#22680=DIRECTION ( 'NONE',  ( 1.000000000000000000, -0.000000000000000000, -1.047444401652940007E-14 ) ) ;
#22683=ADVANCED_FACE ( 'NONE', ( #18609 ), #13203, .F. ) ;
#22684=AXIS2_PLACEMENT_3D ( 'NONE', #20335, #30107, #13477 ) ;
#22761=CARTESIAN_POINT ( 'NONE',  ( 63.50000000000000000, -0.8382352941176473005, -2.222158093317947003 ) ) ;
#22780=CARTESIAN_POINT ( 'NONE',  ( 59.00000000000004974, 3.520859547548639454E-16, 2.874999999999380940 ) ) ;
#22796=EDGE_CURVE ( 'NONE', #30383, #10286, #4023, .T. ) ;
#22809=ORIENTED_EDGE ( 'NONE', *, *, #19499, .T. ) ;
#22841=DIRECTION ( 'NONE',  ( 0.000000000000000000, -1.000000000000000000, 8.673617379884030739E-15 ) ) ;
#22848=VERTEX_POINT ( 'NONE', #6710 ) ;
#22857=CIRCLE ( 'NONE', #4641, 0.2500000000000002220 ) ;
#22877=DIRECTION ( 'NONE',  ( -1.000000000000000000, -0.000000000000000000, 1.047444401652940007E-14 ) ) ;
#22882=DIRECTION ( 'NONE',  ( 1.000000000000000000, -0.000000000000000000, -1.047444401652940007E-14 ) ) ;
#22887=CARTESIAN_POINT ( 'NONE',  ( 63.50000000000004263, -0.7500000000000000000, 1.988246715072691018 ) ) ;
#22942=CARTESIAN_POINT ( 'NONE',  ( 49.00000000000002132, 1.401298464324817071E-42, -5.132477568099407673E-13 ) ) ;
#22949=CARTESIAN_POINT ( 'NONE',  ( 49.00000000000002132, 5.529431079676072613E-15, -5.132477568099407673E-13 ) ) ;
#22978=TOROIDAL_SURFACE ( 'NONE', #9335, 3.950000000000000178, 0.05000000000000000278 ) ;
#22980=CARTESIAN_POINT ( 'NONE',  ( 69.20000000000004547, 0.6441176470588243497, 1.707553061179923892 ) ) ;
#22985=CARTESIAN_POINT ( 'NONE',  ( 69.25000000000004263, 0.8558823529411765385, 2.268940368965340237 ) ) ;
#22991=CARTESIAN_POINT ( 'NONE',  ( 69.24999999999998579, 4.557543281186736018E-17, -2.729289321882064190 ) ) ;
#22994=EDGE_CURVE ( 'NONE', #28523, #31227, #29570, .T. ) ;
#23067=ORIENTED_EDGE ( 'NONE', *, *, #22994, .F. ) ;
#23116=DIRECTION ( 'NONE',  ( 1.000000000000000000, -0.000000000000000000, -1.047444401652940007E-14 ) ) ;
#23121=AXIS2_PLACEMENT_3D ( 'NONE', #22355, #7940, #21328 ) ;
#23131=CIRCLE ( 'NONE', #7925, 2.374999999999998668 ) ;
#23163=ORIENTED_EDGE ( 'NONE', *, *, #15153, .T. ) ;
#23197=FACE_OUTER_BOUND ( 'NONE', #6023, .T. ) ;
#23202=AXIS2_PLACEMENT_3D ( 'NONE', #22949, #776, #10603 ) ;
#23204=ORIENTED_EDGE ( 'NONE', *, *, #21902, .T. ) ;
#23211=ORIENTED_EDGE ( 'NONE', *, *, #17328, .F. ) ;
#23216=DIRECTION ( 'NONE',  ( 1.000000000000000000, 0.000000000000000000, -1.047444401652940007E-14 ) ) ;
#23249=ADVANCED_FACE ( 'NONE', ( #289 ), #17101, .T. ) ;
#23269=CARTESIAN_POINT ( 'NONE',  ( 68.00000000000000000, -0.7500000000000000000, -2.238246715074068582 ) ) ;
#23305=DIRECTION ( 'NONE',  ( 1.000000000000000000, 0.000000000000000000, -1.047444401652940007E-14 ) ) ;
#23326=DIRECTION ( 'NONE',  ( 1.282749433769087582E-30, 1.000000000000000000, 1.224646799147353207E-16 ) ) ;
#23338=CARTESIAN_POINT ( 'NONE',  ( 68.00000000000007105, 1.401298464324817071E-42, 3.499999999999288569 ) ) ;
#23413=DIRECTION ( 'NONE',  ( 1.282749433769087582E-30, 1.000000000000000000, 1.224646799147353207E-16 ) ) ;
#23422=ORIENTED_EDGE ( 'NONE', *, *, #26274, .T. ) ;
#23439=CARTESIAN_POINT ( 'NONE',  ( 49.05000000000005400, 1.401298464324817071E-42, 2.674999999999485123 ) ) ;
#23457=DIRECTION ( 'NONE',  ( -1.047444401652940007E-14, 0.000000000000000000, -1.000000000000000000 ) ) ;
#23471=DIRECTION ( 'NONE',  ( 1.000000000000000000, 0.000000000000000000, -1.047444401652940007E-14 ) ) ;
#23474=DIRECTION ( 'NONE',  ( 0.000000000000000000, 0.000000000000000000, -1.000000000000000000 ) ) ;
#23486=CARTESIAN_POINT ( 'NONE',  ( 63.50000000000000000, -0.7500000000000000000, -1.988246715074021731 ) ) ;
#23502=AXIS2_PLACEMENT_3D ( 'NONE', #3548, #18273, #25698 ) ;
#23508=TOROIDAL_SURFACE ( 'NONE', #9858, 0.3000000000000000444, 0.05000000000000000278 ) ;
#23510=EDGE_LOOP ( 'NONE', ( #21218, #7249, #25302, #26176 ) ) ;
#23523=CARTESIAN_POINT ( 'NONE',  ( 63.50000000000004263, 0.8382352941176473005, 2.222158093316616068 ) ) ;
#23529=VECTOR ( 'NONE', #10674, 1000.000000000000000 ) ;
#23530=VERTEX_POINT ( 'NONE', #4825 ) ;
#23551=CARTESIAN_POINT ( 'NONE',  ( 68.04999999999998295, 1.401298464324817071E-42, -4.000000000000713207 ) ) ;
#23562=TOROIDAL_SURFACE ( 'NONE', #29120, 2.424999999999998934, 0.05000000000000000278 ) ;
#23579=EDGE_LOOP ( 'NONE', ( #12607, #19946, #21521, #28789 ) ) ;
#23589=DIRECTION ( 'NONE',  ( -1.000000000000000000, 0.000000000000000000, 1.047444401652940007E-14 ) ) ;
#23604=CARTESIAN_POINT ( 'NONE',  ( 69.20000000000001705, 0.7500000000000000000, -1.988246715074081017 ) ) ;
#23619=CIRCLE ( 'NONE', #27651, 0.05000000000000012768 ) ;
#23644=CIRCLE ( 'NONE', #24141, 4.000000000000000000 ) ;
#23657=LINE ( 'NONE', #11609, #9932 ) ;
#23670=CYLINDRICAL_SURFACE ( 'NONE', #18368, 1.875000000000000000 ) ;
#23725=FACE_OUTER_BOUND ( 'NONE', #10324, .T. ) ;
#23742=ADVANCED_FACE ( 'NONE', ( #23197 ), #18286, .F. ) ;
#23750=VERTEX_POINT ( 'NONE', #6095 ) ;
#23754=CARTESIAN_POINT ( 'NONE',  ( 68.00000000000004263, 0.6617647058823536987, 1.754335336828722003 ) ) ;
#23762=DIRECTION ( 'NONE',  ( 0.000000000000000000, -0.3529411764705882026, 0.9356455129756979794 ) ) ;
#23765=DIRECTION ( 'NONE',  ( -1.168655815394902336E-14, 0.000000000000000000, -1.000000000000000000 ) ) ;
#23786=VERTEX_POINT ( 'NONE', #1173 ) ;
#23790=DIRECTION ( 'NONE',  ( -1.000000000000000000, 0.000000000000000000, 1.047444401652940007E-14 ) ) ;
#23792=SURFACE_SIDE_STYLE ('',( #2565 ) ) ;
#23799=FACE_BOUND ( 'NONE', #1963, .T. ) ;
#23801=LINE ( 'NONE', #15061, #24644 ) ;
#23818=ADVANCED_FACE ( 'NONE', ( #20969, #30602 ), #13339, .F. ) ;
#23868=CARTESIAN_POINT ( 'NONE',  ( 68.00000000000004263, 0.7500000000000000000, 1.988246715072646387 ) ) ;
#23872=TOROIDAL_SURFACE ( 'NONE', #1094, 2.674999999999998934, 0.05000000000000000278 ) ;
#23903=EDGE_CURVE ( 'NONE', #24785, #25198, #15823, .T. ) ;
#23912=LINE ( 'NONE', #2205, #28569 ) ;
#23913=ADVANCED_FACE ( 'NONE', ( #11627 ), #23670, .T. ) ;
#23932=DIRECTION ( 'NONE',  ( 0.000000000000000000, -3.469446951953614189E-15, 1.000000000000000000 ) ) ;
#23956=DIRECTION ( 'NONE',  ( 1.000000000000000000, -0.000000000000000000, -1.047444401652940007E-14 ) ) ;
#23970=CIRCLE ( 'NONE', #3232, 3.950000000000000178 ) ;
#23980=CYLINDRICAL_SURFACE ( 'NONE', #4978, 0.2500000000000000000 ) ;
#23985=DIRECTION ( 'NONE',  ( -1.000000000000000000, -0.000000000000000000, 1.047444401652940007E-14 ) ) ;
#23987=VERTEX_POINT ( 'NONE', #5589 ) ;
#24036=ORIENTED_EDGE ( 'NONE', *, *, #11732, .F. ) ;
#24041=EDGE_LOOP ( 'NONE', ( #6436, #9584, #11965, #13348 ) ) ;
#24043=DIRECTION ( 'NONE',  ( 1.000000000000000000, 0.000000000000000000, -1.047444401652940007E-14 ) ) ;
#24064=DIRECTION ( 'NONE',  ( 1.000000000000000000, -0.000000000000000000, -1.047444401652940007E-14 ) ) ;
#24087=MECHANICAL_DESIGN_GEOMETRIC_PRESENTATION_REPRESENTATION('',(#7402),#11970);
#24108=AXIS2_PLACEMENT_3D ( 'NONE', #28661, #26435, #23762 ) ;
#24109=AXIS2_PLACEMENT_3D ( 'NONE', #13791, #16684, #23474 ) ;
#24130=DIRECTION ( 'NONE',  ( -1.110223024625156540E-14, 0.000000000000000000, -1.000000000000000000 ) ) ;
#24141=AXIS2_PLACEMENT_3D ( 'NONE', #16318, #14089, #1728 ) ;
#24145=ADVANCED_FACE ( 'NONE', ( #6062 ), #17960, .T. ) ;
#24210=DIRECTION ( 'NONE',  ( 1.000000000000000000, -0.000000000000000000, -1.047444401652940007E-14 ) ) ;
#24219=CIRCLE ( 'NONE', #6004, 0.2499999999999997780 ) ;
#24226=EDGE_CURVE ( 'NONE', #31054, #1785, #28581, .T. ) ;
#24263=DIRECTION ( 'NONE',  ( 0.000000000000000000, 0.000000000000000000, -1.000000000000000000 ) ) ;
#24267=DIRECTION ( 'NONE',  ( 1.000000000000000000, -0.000000000000000000, -1.047444401652940007E-14 ) ) ;
#24278=CARTESIAN_POINT ( 'NONE',  ( 63.50000000000002842, 1.401298464324817071E-42, -6.651271950496169736E-13 ) ) ;
#24281=AXIS2_PLACEMENT_3D ( 'NONE', #19276, #4681, #12419 ) ;
#24329=CIRCLE ( 'NONE', #14712, 4.000000000000000000 ) ;
#24333=EDGE_CURVE ( 'NONE', #15675, #865, #258, .T. ) ;
#24359=CARTESIAN_POINT ( 'NONE',  ( 69.23535533905932482, 3.976613875667303688E-16, -2.764644660941391052 ) ) ;
#24361=ORIENTED_EDGE ( 'NONE', *, *, #2155, .T. ) ;
#24380=DIRECTION ( 'NONE',  ( 1.189524669241238948E-14, 0.000000000000000000, 1.000000000000000000 ) ) ;
#24395=DIRECTION ( 'NONE',  ( -7.401486830834382195E-15, 0.000000000000000000, -1.000000000000000000 ) ) ;
#24431=VERTEX_POINT ( 'NONE', #22343 ) ;
#24446=EDGE_CURVE ( 'NONE', #25040, #28523, #13362, .T. ) ;
#24481=ORIENTED_EDGE ( 'NONE', *, *, #3844, .T. ) ;
#24482=LINE ( 'NONE', #2792, #22538 ) ;
#24484=FACE_OUTER_BOUND ( 'NONE', #24648, .T. ) ;
#24487=ORIENTED_EDGE ( 'NONE', *, *, #670, .F. ) ;
#24504=EDGE_CURVE ( 'NONE', #1976, #27508, #4314, .T. ) ;
#24506=CARTESIAN_POINT ( 'NONE',  ( 48.99999999999999289, 1.401298464324817071E-42, -2.875000000000512035 ) ) ;
#24510=AXIS2_PLACEMENT_3D ( 'NONE', #14393, #24064, #25419 ) ;
#24521=CARTESIAN_POINT ( 'NONE',  ( 69.25000000000004263, -0.7500000000000000000, 1.988246715072632620 ) ) ;
#24542=VERTEX_POINT ( 'NONE', #1793 ) ;
#24558=FACE_OUTER_BOUND ( 'NONE', #14278, .T. ) ;
#24578=AXIS2_PLACEMENT_3D ( 'NONE', #14981, #30011, #7849 ) ;
#24590=CARTESIAN_POINT ( 'NONE',  ( 58.99999999999998579, 1.401298464324817071E-42, -4.000000000000617284 ) ) ;
#24596=CIRCLE ( 'NONE', #12949, 0.05000000000000012768 ) ;
#24597=DIRECTION ( 'NONE',  ( 1.000000000000000000, -0.000000000000000000, -1.047444401652940007E-14 ) ) ;
#24603=( LENGTH_UNIT ( ) NAMED_UNIT ( * ) SI_UNIT ( .MILLI., .METRE. ) );
#24604=DIRECTION ( 'NONE',  ( 1.156482317317871449E-14, 0.000000000000000000, 1.000000000000000000 ) ) ;
#24625=EDGE_CURVE ( 'NONE', #1785, #31054, #3304, .T. ) ;
#24641=CARTESIAN_POINT ( 'NONE',  ( 69.20000000000003126, 1.401298464324817071E-42, -7.248315259438346108E-13 ) ) ;
#24644=VECTOR ( 'NONE', #26931, 1000.000000000000000 ) ;
#24648=EDGE_LOOP ( 'NONE', ( #27924, #26463, #8147, #19653 ) ) ;
#24669=CARTESIAN_POINT ( 'NONE',  ( 69.25000000000004263, 0.7500000000000000000, 1.988246715072633064 ) ) ;
#24679=CIRCLE ( 'NONE', #5473, 0.2500000000000002220 ) ;
#24690=CARTESIAN_POINT ( 'NONE',  ( 49.05000000000005400, 1.401298464324817071E-42, 2.824999999999485034 ) ) ;
#24728=EDGE_CURVE ( 'NONE', #23987, #12273, #5306, .T. ) ;
#24737=ORIENTED_EDGE ( 'NONE', *, *, #1434, .F. ) ;
#24762=ADVANCED_FACE ( 'NONE', ( #20759 ), #277, .T. ) ;
#24778=ORIENTED_EDGE ( 'NONE', *, *, #27819, .F. ) ;
#24785=VERTEX_POINT ( 'NONE', #1254 ) ;
#24810=CARTESIAN_POINT ( 'NONE',  ( 68.00000000000002842, 1.401298464324817071E-42, -7.122621931239993559E-13 ) ) ;
#24854=DIRECTION ( 'NONE',  ( 0.000000000000000000, -7.228014483236697541E-16, -1.000000000000000000 ) ) ;
#24877=FACE_OUTER_BOUND ( 'NONE', #20267, .T. ) ;
#24893=CARTESIAN_POINT ( 'NONE',  ( 69.25000000000000000, 0.6441176470588245717, -1.707553061181374732 ) ) ;
#24915=VERTEX_POINT ( 'NONE', #30868 ) ;
#24938=CARTESIAN_POINT ( 'NONE',  ( 69.05000000000002558, 4.557543281186736018E-17, -7.232603593413552923E-13 ) ) ;
#24941=CIRCLE ( 'NONE', #20415, 0.04999999999999994033 ) ;
#24986=ORIENTED_EDGE ( 'NONE', *, *, #7209, .T. ) ;
#24997=CARTESIAN_POINT ( 'NONE',  ( 68.00000000000001421, 1.401298464324817071E-42, -7.122621931239992550E-13 ) ) ;
#25001=CARTESIAN_POINT ( 'NONE',  ( 68.05000000000002558, 1.401298464324817071E-42, -7.127859153248258291E-13 ) ) ;
#25003=EDGE_CURVE ( 'NONE', #3817, #5818, #5672, .T. ) ;
#25015=DIRECTION ( 'NONE',  ( 9.297243531610763781E-15, 0.000000000000000000, 1.000000000000000000 ) ) ;
#25027=FACE_OUTER_BOUND ( 'NONE', #924, .T. ) ;
#25040=VERTEX_POINT ( 'NONE', #12631 ) ;
#25071=AXIS2_PLACEMENT_3D ( 'NONE', #23439, #28346, #6498 ) ;
#25083=VERTEX_POINT ( 'NONE', #12315 ) ;
#25084=CIRCLE ( 'NONE', #5381, 0.2999999999999999334 ) ;
#25091=DIRECTION ( 'NONE',  ( -1.000000000000000000, 0.000000000000000000, 1.047444401652940007E-14 ) ) ;
#25099=DIRECTION ( 'NONE',  ( -1.282749433769087582E-30, 1.000000000000000000, -1.224646799147353207E-16 ) ) ;
#25111=AXIS2_PLACEMENT_3D ( 'NONE', #17949, #13645, #8894 ) ;
#25130=AXIS2_PLACEMENT_3D ( 'NONE', #27737, #3811, #6347 ) ;
#25131=ORIENTED_EDGE ( 'NONE', *, *, #22571, .F. ) ;
#25132=DIRECTION ( 'NONE',  ( -1.054009200593503061E-14, 0.000000000000000000, -1.000000000000000000 ) ) ;
#25139=DIRECTION ( 'NONE',  ( -1.000000000000000000, 0.000000000000000000, 1.047444401652940007E-14 ) ) ;
#25145=AXIS2_PLACEMENT_3D ( 'NONE', #14553, #18845, #31177 ) ;
#25153=VECTOR ( 'NONE', #26605, 1000.000000000000000 ) ;
#25163=AXIS2_PLACEMENT_3D ( 'NONE', #6735, #4824, #2296 ) ;
#25198=VERTEX_POINT ( 'NONE', #23551 ) ;
#25220=ORIENTED_EDGE ( 'NONE', *, *, #19355, .T. ) ;
#25250=DIRECTION ( 'NONE',  ( 0.000000000000000000, 0.000000000000000000, 1.000000000000000000 ) ) ;
#25262=FACE_OUTER_BOUND ( 'NONE', #6248, .T. ) ;
#25266=CARTESIAN_POINT ( 'NONE',  ( 64.99999999999998579, 1.401298464324817071E-42, -3.950000000000681410 ) ) ;
#25293=CARTESIAN_POINT ( 'NONE',  ( 69.20000000000001705, 0.5000000000000000000, -1.988246715074081017 ) ) ;
#25299=DIRECTION ( 'NONE',  ( 0.000000000000000000, 0.000000000000000000, -1.000000000000000000 ) ) ;
#25301=ADVANCED_FACE ( 'NONE', ( #13332 ), #1779, .T. ) ;
#25302=ORIENTED_EDGE ( 'NONE', *, *, #17782, .F. ) ;
#25318=UNCERTAINTY_MEASURE_WITH_UNIT (LENGTH_MEASURE( 1.000000000000000082E-05 ), #9836, 'distance_accuracy_value', 'NONE');
#25336=ADVANCED_FACE ( 'NONE', ( #29982 ), #19234, .T. ) ;
#25360=DIRECTION ( 'NONE',  ( 9.188425696205898615E-15, 0.000000000000000000, 1.000000000000000000 ) ) ;
#25370=DIRECTION ( 'NONE',  ( 1.047444401652940007E-14, 0.000000000000000000, 1.000000000000000000 ) ) ;
#25381=CARTESIAN_POINT ( 'NONE',  ( 69.04999999999999716, 4.155057991226904698E-16, -3.020710678119369330 ) ) ;
#25385=CYLINDRICAL_SURFACE ( 'NONE', #26118, 4.000000000000000000 ) ;
#25392=DIRECTION ( 'NONE',  ( -1.000000000000000000, 0.000000000000000000, 1.047444401652940007E-14 ) ) ;
#25402=EDGE_LOOP ( 'NONE', ( #15017, #21670, #4339, #25131 ) ) ;
#25415=CARTESIAN_POINT ( 'NONE',  ( 69.20000000000001705, -0.7500000000000000000, -1.988246715074081017 ) ) ;
#25419=DIRECTION ( 'NONE',  ( 0.000000000000000000, -3.469446951953614189E-15, 1.000000000000000000 ) ) ;
#25421=DIRECTION ( 'NONE',  ( 1.156482317317871449E-14, 0.000000000000000000, 1.000000000000000000 ) ) ;
#25470=DIRECTION ( 'NONE',  ( -1.000000000000000000, 0.000000000000000000, 1.047444401652940007E-14 ) ) ;
#25539=EDGE_CURVE ( 'NONE', #1752, #27301, #24596, .T. ) ;
#25569=CIRCLE ( 'NONE', #9898, 0.2999999999999999334 ) ;
#25591=CIRCLE ( 'NONE', #13433, 0.2500000000000000000 ) ;
#25604=CIRCLE ( 'NONE', #6905, 2.674999999999998934 ) ;
#25631=AXIS2_PLACEMENT_3D ( 'NONE', #11911, #26933, #21598 ) ;
#25641=CARTESIAN_POINT ( 'NONE',  ( 69.25000000000000000, -0.7500000000000000000, -1.988246715074081905 ) ) ;
#25657=DIRECTION ( 'NONE',  ( 1.057355261547768637E-14, 0.000000000000000000, 1.000000000000000000 ) ) ;
#25685=ORIENTED_EDGE ( 'NONE', *, *, #13535, .F. ) ;
#25695=CIRCLE ( 'NONE', #18124, 3.950000000000000178 ) ;
#25698=DIRECTION ( 'NONE',  ( 9.654113257610060303E-15, 0.000000000000000000, 1.000000000000000000 ) ) ;
#25699=DIRECTION ( 'NONE',  ( 1.000000000000000000, 0.000000000000000000, -1.047444401652940007E-14 ) ) ;
#25706=FACE_OUTER_BOUND ( 'NONE', #22375, .T. ) ;
#25709=ORIENTED_EDGE ( 'NONE', *, *, #26274, .F. ) ;
#25724=DIRECTION ( 'NONE',  ( -7.604267291953133322E-15, 0.000000000000000000, -1.000000000000000000 ) ) ;
#25731=DIRECTION ( 'NONE',  ( -1.000000000000000000, 0.000000000000000000, 1.047444401652940007E-14 ) ) ;
#25779=CARTESIAN_POINT ( 'NONE',  ( 60.67929986713512136, 3.641481190980049571E-16, -2.973495046503342287 ) ) ;
#25805=EDGE_LOOP ( 'NONE', ( #16450, #14919 ) ) ;
#25827=CARTESIAN_POINT ( 'NONE',  ( 69.20000000000005969, 0.7500000000000000000, 1.988246715072633952 ) ) ;
#25840=EDGE_CURVE ( 'NONE', #23987, #10712, #21574, .T. ) ;
#25844=DIRECTION ( 'NONE',  ( 1.000000000000000000, -0.000000000000000000, -1.047444401652940007E-14 ) ) ;
#25849=MANIFOLD_SOLID_BREP ( 'Stock-MAS-683-1', #868 ) ;
#25881=DIRECTION ( 'NONE',  ( -1.000000000000000000, 0.000000000000000000, 1.047444401652940007E-14 ) ) ;
#25891=CIRCLE ( 'NONE', #16294, 0.05000000000000012768 ) ;
#25899=ORIENTED_EDGE ( 'NONE', *, *, #23903, .F. ) ;
#25910=ORIENTED_EDGE ( 'NONE', *, *, #15854, .F. ) ;
#25927=DIRECTION ( 'NONE',  ( -1.000000000000000000, -0.000000000000000000, 1.047444401652940007E-14 ) ) ;
#25942=CARTESIAN_POINT ( 'NONE',  ( 49.05000000000002558, 1.401298464324817071E-42, -5.137714790107672405E-13 ) ) ;
#25987=CARTESIAN_POINT ( 'NONE',  ( 0.000000000000000000, 0.000000000000000000, 0.000000000000000000 ) ) ;
#25990=ORIENTED_EDGE ( 'NONE', *, *, #10190, .T. ) ;
#25994=DIRECTION ( 'NONE',  ( 0.000000000000000000, 0.000000000000000000, 1.000000000000000000 ) ) ;
#26005=TOROIDAL_SURFACE ( 'NONE', #12354, 0.3000000000000000444, 0.05000000000000000278 ) ;
#26014=DIRECTION ( 'NONE',  ( 1.000000000000000000, -0.000000000000000000, -1.047444401652940007E-14 ) ) ;
#26036=DIRECTION ( 'NONE',  ( 1.047444401652940007E-14, 0.000000000000000000, 1.000000000000000000 ) ) ;
#26050=AXIS2_PLACEMENT_3D ( 'NONE', #10637, #5416, #20314 ) ;
#26053=VERTEX_POINT ( 'NONE', #16352 ) ;
#26065=TOROIDAL_SURFACE ( 'NONE', #12403, 2.824999999999998845, 0.05000000000000000278 ) ;
#26095=ORIENTED_EDGE ( 'NONE', *, *, #10974, .T. ) ;
#26118=AXIS2_PLACEMENT_3D ( 'NONE', #30435, #25699, #4006 ) ;
#26125=EDGE_CURVE ( 'NONE', #27518, #26053, #20600, .T. ) ;
#26153=( NAMED_UNIT ( * ) SI_UNIT ( $, .STERADIAN. ) SOLID_ANGLE_UNIT ( ) );
#26176=ORIENTED_EDGE ( 'NONE', *, *, #15172, .F. ) ;
#26181=ORIENTED_EDGE ( 'NONE', *, *, #859, .F. ) ;
#26197=ORIENTED_EDGE ( 'NONE', *, *, #2052, .F. ) ;
#26214=CARTESIAN_POINT ( 'NONE',  ( 63.50000000000000000, -0.7500000000000000000, -2.238246715074021953 ) ) ;
#26219=VERTEX_POINT ( 'NONE', #29456 ) ;
#26274=EDGE_CURVE ( 'NONE', #30539, #27301, #19606, .T. ) ;
#26304=DIRECTION ( 'NONE',  ( 1.000000000000000000, -0.000000000000000000, -1.047444401652940007E-14 ) ) ;
#26310=EDGE_CURVE ( 'NONE', #10286, #24915, #7974, .T. ) ;
#26323=DIRECTION ( 'NONE',  ( 1.000000000000000000, -0.000000000000000000, -1.047444401652940007E-14 ) ) ;
#26361=DIRECTION ( 'NONE',  ( -1.000000000000000000, 0.000000000000000000, 1.047444401652940007E-14 ) ) ;
#26372=EDGE_LOOP ( 'NONE', ( #25220, #29377, #21586, #20474 ) ) ;
#26397=FACE_OUTER_BOUND ( 'NONE', #13121, .T. ) ;
#26411=DIRECTION ( 'NONE',  ( 1.057355261547768637E-14, 0.000000000000000000, 1.000000000000000000 ) ) ;
#26425=CARTESIAN_POINT ( 'NONE',  ( 68.00000000000001421, 1.401298464324817071E-42, -7.122621931239992550E-13 ) ) ;
#26435=DIRECTION ( 'NONE',  ( -3.696862594069201137E-15, -0.9356455129756980904, -0.3529411764705883137 ) ) ;
#26445=CARTESIAN_POINT ( 'NONE',  ( 69.00000000000001421, 1.401298464324817071E-42, -7.227366371405287181E-13 ) ) ;
#26463=ORIENTED_EDGE ( 'NONE', *, *, #17141, .T. ) ;
#26476=EDGE_CURVE ( 'NONE', #27301, #30539, #23644, .T. ) ;
#26483=EDGE_CURVE ( 'NONE', #865, #171, #11997, .T. ) ;
#26489=EDGE_LOOP ( 'NONE', ( #5127, #2558, #20509, #11028 ) ) ;
#26517=DIRECTION ( 'NONE',  ( 1.000000000000000000, -0.000000000000000000, -1.047444401652940007E-14 ) ) ;
#26520=CIRCLE ( 'NONE', #10334, 2.374999999999998668 ) ;
#26534=ORIENTED_EDGE ( 'NONE', *, *, #9489, .T. ) ;
#26564=ORIENTED_EDGE ( 'NONE', *, *, #8165, .F. ) ;
#26605=DIRECTION ( 'NONE',  ( 1.000000000000000000, -0.000000000000000000, -1.047444401652940007E-14 ) ) ;
#26651=AXIS2_PLACEMENT_3D ( 'NONE', #12506, #7616, #29595 ) ;
#26654=FACE_BOUND ( 'NONE', #27858, .T. ) ;
#26668=CIRCLE ( 'NONE', #23121, 1.824999999999999956 ) ;
#26705=CIRCLE ( 'NONE', #30734, 3.950000000000000178 ) ;
#26713=ORIENTED_EDGE ( 'NONE', *, *, #10288, .T. ) ;
#26714=DIRECTION ( 'NONE',  ( -1.000000000000000000, 0.000000000000000000, 1.047444401652940007E-14 ) ) ;
#26761=EDGE_CURVE ( 'NONE', #6108, #28026, #29678, .T. ) ;
#26763=CARTESIAN_POINT ( 'NONE',  ( 49.00000000000004974, 1.401298464324817071E-42, 2.674999999999486011 ) ) ;
#26769=ORIENTED_EDGE ( 'NONE', *, *, #30850, .F. ) ;
#26776=CARTESIAN_POINT ( 'NONE',  ( 68.00000000000000000, 0.7500000000000000000, -1.988246715074068582 ) ) ;
#26791=FACE_OUTER_BOUND ( 'NONE', #2798, .T. ) ;
#26830=DIRECTION ( 'NONE',  ( 0.000000000000000000, -1.224646799147353207E-16, 1.000000000000000000 ) ) ;
#26856=CARTESIAN_POINT ( 'NONE',  ( 69.25000000000004263, 4.557543281186736018E-17, 2.749999999999274358 ) ) ;
#26922=EDGE_CURVE ( 'NONE', #29622, #26053, #30806, .T. ) ;
#26931=DIRECTION ( 'NONE',  ( -1.000000000000000000, 0.000000000000000000, 1.047444401652940007E-14 ) ) ;
#26933=DIRECTION ( 'NONE',  ( -1.000000000000000000, 0.000000000000000000, 1.047444401652940007E-14 ) ) ;
#26937=DIRECTION ( 'NONE',  ( 0.000000000000000000, 2.529805069132844337E-15, -1.000000000000000000 ) ) ;
#26947=ORIENTED_EDGE ( 'NONE', *, *, #26761, .T. ) ;
#26956=ADVANCED_FACE ( 'NONE', ( #4522, #19266 ), #30963, .T. ) ;
#26964=ORIENTED_EDGE ( 'NONE', *, *, #19144, .T. ) ;
#27047=EDGE_CURVE ( 'NONE', #9761, #22848, #12440, .T. ) ;
#27052=DIRECTION ( 'NONE',  ( 1.000000000000000000, 0.000000000000000000, -1.047444401652940007E-14 ) ) ;
#27070=CIRCLE ( 'NONE', #7379, 2.424999999999998934 ) ;
#27079=EDGE_CURVE ( 'NONE', #5843, #6314, #19869, .T. ) ;
#27082=FACE_OUTER_BOUND ( 'NONE', #15242, .T. ) ;
#27088=DIRECTION ( 'NONE',  ( -1.000000000000000000, 0.000000000000000000, 1.047444401652940007E-14 ) ) ;
#27093=EDGE_CURVE ( 'NONE', #14020, #12243, #18027, .T. ) ;
#27105=AXIS2_PLACEMENT_3D ( 'NONE', #27745, #3531, #8424 ) ;
#27119=DIRECTION ( 'NONE',  ( 1.000000000000000000, 0.000000000000000000, -1.047444401652940007E-14 ) ) ;
#27168=AXIS2_PLACEMENT_3D ( 'NONE', #24278, #7642, #2591 ) ;
#27191=ORIENTED_EDGE ( 'NONE', *, *, #28420, .F. ) ;
#27194=DIRECTION ( 'NONE',  ( -1.047444401652940007E-14, 0.000000000000000000, -1.000000000000000000 ) ) ;
#27205=DIRECTION ( 'NONE',  ( 1.189524669241239105E-14, 0.000000000000000000, 1.000000000000000000 ) ) ;
#27213=AXIS2_PLACEMENT_3D ( 'NONE', #30945, #7199, #9590 ) ;
#27231=ORIENTED_EDGE ( 'NONE', *, *, #2155, .F. ) ;
#27275=ORIENTED_EDGE ( 'NONE', *, *, #4003, .F. ) ;
#27295=DIRECTION ( 'NONE',  ( 1.000000000000000000, -0.000000000000000000, -1.047444401652940007E-14 ) ) ;
#27301=VERTEX_POINT ( 'NONE', #20806 ) ;
#27304=TOROIDAL_SURFACE ( 'NONE', #523, 2.824999999999998845, 0.05000000000000000278 ) ;
#27339=VERTEX_POINT ( 'NONE', #4158 ) ;
#27365=ORIENTED_EDGE ( 'NONE', *, *, #3117, .F. ) ;
#27370=CARTESIAN_POINT ( 'NONE',  ( 68.00000000000000000, 0.7500000000000000000, -2.238246715074068582 ) ) ;
#27384=EDGE_LOOP ( 'NONE', ( #30182, #18316, #23067, #20684 ) ) ;
#27409=CARTESIAN_POINT ( 'NONE',  ( 64.94999999999997442, 1.401298464324817071E-42, -4.000000000000680345 ) ) ;
#27426=ORIENTED_EDGE ( 'NONE', *, *, #21414, .T. ) ;
#27481=CARTESIAN_POINT ( 'NONE',  ( 60.67929986713517820, 1.401298464324817071E-42, 2.973495046502070860 ) ) ;
#27484=ORIENTED_EDGE ( 'NONE', *, *, #27047, .F. ) ;
#27490=ORIENTED_EDGE ( 'NONE', *, *, #29506, .F. ) ;
#27508=VERTEX_POINT ( 'NONE', #27409 ) ;
#27509=EDGE_CURVE ( 'NONE', #25040, #21014, #340, .T. ) ;
#27518=VERTEX_POINT ( 'NONE', #5884 ) ;
#27526=ORIENTED_EDGE ( 'NONE', *, *, #7513, .F. ) ;
#27527=EDGE_LOOP ( 'NONE', ( #11452, #16020 ) ) ;
#27541=ORIENTED_EDGE ( 'NONE', *, *, #20362, .T. ) ;
#27572=ADVANCED_FACE ( 'NONE', ( #27730 ), #18050, .T. ) ;
#27590=CARTESIAN_POINT ( 'NONE',  ( 69.20000000000005969, 0.5000000000000000000, 1.988246715072633952 ) ) ;
#27597=AXIS2_PLACEMENT_3D ( 'NONE', #8456, #25392, #20670 ) ;
#27651=AXIS2_PLACEMENT_3D ( 'NONE', #25381, #23326, #8281 ) ;
#27661=CIRCLE ( 'NONE', #26651, 0.2499999999999997780 ) ;
#27662=VERTEX_POINT ( 'NONE', #1912 ) ;
#27677=AXIS2_PLACEMENT_3D ( 'NONE', #4880, #24210, #17095 ) ;
#27680=AXIS2_PLACEMENT_3D ( 'NONE', #3797, #9199, #6335 ) ;
#27696=ORIENTED_EDGE ( 'NONE', *, *, #15624, .F. ) ;
#27697=FACE_OUTER_BOUND ( 'NONE', #8421, .T. ) ;
#27708=EDGE_CURVE ( 'NONE', #2745, #5953, #13918, .T. ) ;
#27721=DIRECTION ( 'NONE',  ( -1.047444401652940007E-14, 0.000000000000000000, -1.000000000000000000 ) ) ;
#27723=DIRECTION ( 'NONE',  ( -1.040834085586084257E-14, 0.000000000000000000, -1.000000000000000000 ) ) ;
#27727=CIRCLE ( 'NONE', #22684, 0.04999999999999449329 ) ;
#27730=FACE_OUTER_BOUND ( 'NONE', #13945, .T. ) ;
#27737=CARTESIAN_POINT ( 'NONE',  ( 59.00000000000002132, 1.401298464324817071E-42, -6.179921969752347932E-13 ) ) ;
#27745=CARTESIAN_POINT ( 'NONE',  ( 69.20000000000004547, 0.7500000000000000000, 1.988246715072631732 ) ) ;
#27771=DIRECTION ( 'NONE',  ( 0.000000000000000000, 0.000000000000000000, -1.000000000000000000 ) ) ;
#27785=ORIENTED_EDGE ( 'NONE', *, *, #25003, .T. ) ;
#27819=EDGE_CURVE ( 'NONE', #31054, #24915, #20092, .T. ) ;
#27858=EDGE_LOOP ( 'NONE', ( #14765, #29503 ) ) ;
#27904=VERTEX_POINT ( 'NONE', #3000 ) ;
#27923=EDGE_CURVE ( 'NONE', #5901, #21780, #9678, .T. ) ;
#27924=ORIENTED_EDGE ( 'NONE', *, *, #24504, .F. ) ;
#27958=EDGE_CURVE ( 'NONE', #590, #29022, #17041, .T. ) ;
#27979=CARTESIAN_POINT ( 'NONE',  ( 69.20000000000001705, 0.7500000000000000000, -2.238246715074081017 ) ) ;
#27988=CARTESIAN_POINT ( 'NONE',  ( 69.20000000000001705, -0.6617647058823530326, -1.754335336830158631 ) ) ;
#28007=CARTESIAN_POINT ( 'NONE',  ( 49.00000000000002132, 1.401298464324817071E-42, -5.132477568099407673E-13 ) ) ;
#28009=DIRECTION ( 'NONE',  ( -1.000000000000000000, 0.000000000000000000, 1.047444401652940007E-14 ) ) ;
#28013=CARTESIAN_POINT ( 'NONE',  ( 69.20000000000001705, 0.7500000000000000000, -1.988246715074081017 ) ) ;
#28023=CARTESIAN_POINT ( 'NONE',  ( 49.05000000000002558, 1.401298464324817071E-42, -5.137714790107672405E-13 ) ) ;
#28026=VERTEX_POINT ( 'NONE', #21048 ) ;
#28038=ORIENTED_EDGE ( 'NONE', *, *, #18457, .F. ) ;
#28070=CARTESIAN_POINT ( 'NONE',  ( 69.25000000000000000, -0.7500000000000000000, -1.988246715074081905 ) ) ;
#28081=EDGE_LOOP ( 'NONE', ( #9271, #12735, #13266, #27526 ) ) ;
#28111=EDGE_LOOP ( 'NONE', ( #14303, #11139 ) ) ;
#28162=EDGE_CURVE ( 'NONE', #14417, #6108, #12485, .T. ) ;
#28179=ORIENTED_EDGE ( 'NONE', *, *, #27819, .T. ) ;
#28212=AXIS2_PLACEMENT_3D ( 'NONE', #17688, #2788, #29705 ) ;
#28213=ORIENTED_EDGE ( 'NONE', *, *, #12959, .F. ) ;
#28215=DIRECTION ( 'NONE',  ( 1.000000000000000000, 0.000000000000000000, -1.047444401652940007E-14 ) ) ;
#28243=DIRECTION ( 'NONE',  ( 0.000000000000000000, -1.000000000000000000, 0.000000000000000000 ) ) ;
#28247=DIRECTION ( 'NONE',  ( 1.000000000000000000, 0.000000000000000000, -1.047444401652940007E-14 ) ) ;
#28249=ORIENTED_EDGE ( 'NONE', *, *, #24728, .F. ) ;
#28276=AXIS2_PLACEMENT_3D ( 'NONE', #17619, #7497, #12538 ) ;
#28313=ADVANCED_FACE ( 'NONE', ( #4959, #26654 ), #512, .T. ) ;
#28316=FACE_OUTER_BOUND ( 'NONE', #5443, .T. ) ;
#28330=AXIS2_PLACEMENT_3D ( 'NONE', #15438, #25091, #13063 ) ;
#28346=DIRECTION ( 'NONE',  ( 0.000000000000000000, -1.000000000000000000, 0.000000000000000000 ) ) ;
#28353=DIRECTION ( 'NONE',  ( 1.000000000000000000, -0.000000000000000000, -1.047444401652940007E-14 ) ) ;
#28386=DIRECTION ( 'NONE',  ( -1.016952486242704214E-14, 0.000000000000000000, -1.000000000000000000 ) ) ;
#28410=VECTOR ( 'NONE', #22586, 1000.000000000000114 ) ;
#28420=EDGE_CURVE ( 'NONE', #5818, #5953, #4932, .T. ) ;
#28436=ORIENTED_EDGE ( 'NONE', *, *, #9443, .T. ) ;
#28489=CIRCLE ( 'NONE', #4722, 0.05000000000000002359 ) ;
#28501=ADVANCED_FACE ( 'NONE', ( #16482 ), #9975, .T. ) ;
#28523=VERTEX_POINT ( 'NONE', #2071 ) ;
#28533=FACE_OUTER_BOUND ( 'NONE', #18946, .T. ) ;
#28566=EDGE_CURVE ( 'NONE', #26219, #14020, #16960, .T. ) ;
#28569=VECTOR ( 'NONE', #21551, 1000.000000000000000 ) ;
#28576=ORIENTED_EDGE ( 'NONE', *, *, #1669, .F. ) ;
#28581=CIRCLE ( 'NONE', #18986, 3.020710678118645909 ) ;
#28618=LINE ( 'NONE', #21507, #13466 ) ;
#28622=VECTOR ( 'NONE', #29862, 1000.000000000000000 ) ;
#28634=CONICAL_SURFACE ( 'NONE', #12434, 2.750000000000000000, 0.7853981633974466137 ) ;
#28648=ORIENTED_EDGE ( 'NONE', *, *, #22571, .T. ) ;
#28655=CONICAL_SURFACE ( 'NONE', #14979, 2.750000000000000000, 0.7853981633974466137 ) ;
#28661=CARTESIAN_POINT ( 'NONE',  ( 69.20000000000005969, -0.8558823529411765385, 2.268940368965341126 ) ) ;
#28666=CIRCLE ( 'NONE', #11455, 2.729289321881338548 ) ;
#28687=CARTESIAN_POINT ( 'NONE',  ( 69.20000000000000284, 0.8382352941176473005, -2.222158093318006067 ) ) ;
#28693=DIRECTION ( 'NONE',  ( 1.009293658750142281E-14, 0.000000000000000000, 1.000000000000000000 ) ) ;
#28702=VECTOR ( 'NONE', #592, 1000.000000000000000 ) ;
#28705=CIRCLE ( 'NONE', #31231, 2.374999999999998668 ) ;
#28732=ORIENTED_EDGE ( 'NONE', *, *, #19865, .F. ) ;
#28740=ORIENTED_EDGE ( 'NONE', *, *, #27093, .T. ) ;
#28749=FACE_OUTER_BOUND ( 'NONE', #7340, .T. ) ;
#28789=ORIENTED_EDGE ( 'NONE', *, *, #5935, .T. ) ;
#28799=DIRECTION ( 'NONE',  ( 0.000000000000000000, 0.000000000000000000, -1.000000000000000000 ) ) ;
#28811=DIRECTION ( 'NONE',  ( -1.168655815394902336E-14, 0.000000000000000000, -1.000000000000000000 ) ) ;
#28818=DIRECTION ( 'NONE',  ( 1.000000000000000000, 0.000000000000000000, -1.047444401652940007E-14 ) ) ;
#28830=CARTESIAN_POINT ( 'NONE',  ( 63.50000000000000000, 1.401298464324817071E-42, -2.375000000000663913 ) ) ;
#28831=FACE_OUTER_BOUND ( 'NONE', #16437, .T. ) ;
#28843=CARTESIAN_POINT ( 'NONE',  ( 69.25000000000000000, 0.7500000000000000000, -1.988246715074081905 ) ) ;
#28865=DIRECTION ( 'NONE',  ( 1.000000000000000000, 0.000000000000000000, -1.047444401652940007E-14 ) ) ;
#28868=ADVANCED_FACE ( 'NONE', ( #15140 ), #10521, .T. ) ;
#28871=DIRECTION ( 'NONE',  ( 1.000000000000000000, -0.000000000000000000, -1.047444401652940007E-14 ) ) ;
#28895=EDGE_LOOP ( 'NONE', ( #16504, #25990, #13811, #18104 ) ) ;
#28898=SURFACE_STYLE_USAGE ( .BOTH. , #10345 ) ;
#28920=EDGE_LOOP ( 'NONE', ( #8613, #26564, #3738, #20079 ) ) ;
#28922=DIRECTION ( 'NONE',  ( 1.282749433769087582E-30, 1.000000000000000000, 1.224646799147353207E-16 ) ) ;
#28926=DIRECTION ( 'NONE',  ( -1.016952486242704214E-14, 0.000000000000000000, -1.000000000000000000 ) ) ;
#28927=CIRCLE ( 'NONE', #19336, 2.764644660940665855 ) ;
#28934=ADVANCED_BREP_SHAPE_REPRESENTATION ( '', ( #25849, #9018 ), #21749 ) ;
#28945=EDGE_CURVE ( 'NONE', #20971, #12243, #723, .T. ) ;
#28954=FACE_OUTER_BOUND ( 'NONE', #4451, .T. ) ;
#28963=ORIENTED_EDGE ( 'NONE', *, *, #12188, .F. ) ;
#28995=FILL_AREA_STYLE ('',( #14113 ) ) ;
#29022=VERTEX_POINT ( 'NONE', #23338 ) ;
#29120=AXIS2_PLACEMENT_3D ( 'NONE', #30430, #23471, #18891 ) ;
#29141=ORIENTED_EDGE ( 'NONE', *, *, #17238, .F. ) ;
#29145=AXIS2_PLACEMENT_3D ( 'NONE', #28023, #15995, #25657 ) ;
#29152=EDGE_CURVE ( 'NONE', #14189, #30539, #11535, .T. ) ;
#29167=FACE_OUTER_BOUND ( 'NONE', #12455, .T. ) ;
#29174=DIRECTION ( 'NONE',  ( -3.696862594069201137E-15, 0.9356455129756980904, -0.3529411764705883137 ) ) ;
#29179=DIRECTION ( 'NONE',  ( 0.000000000000000000, 0.3529411764705897014, -0.9356455129756974243 ) ) ;
#29209=AXIS2_PLACEMENT_3D ( 'NONE', #22454, #13094, #19775 ) ;
#29276=AXIS2_PLACEMENT_3D ( 'NONE', #23486, #4014, #27771 ) ;
#29311=ADVANCED_FACE ( 'NONE', ( #3517 ), #19836, .F. ) ;
#29317=CARTESIAN_POINT ( 'NONE',  ( 69.25000000000000000, -0.8558823529411765385, -2.268940368966791077 ) ) ;
#29334=ORIENTED_EDGE ( 'NONE', *, *, #6158, .T. ) ;
#29372=ORIENTED_EDGE ( 'NONE', *, *, #9899, .F. ) ;
#29377=ORIENTED_EDGE ( 'NONE', *, *, #2761, .F. ) ;
#29406=DIRECTION ( 'NONE',  ( 1.000000000000000000, 0.000000000000000000, -1.047444401652940007E-14 ) ) ;
#29416=FACE_OUTER_BOUND ( 'NONE', #27384, .T. ) ;
#29454=DIRECTION ( 'NONE',  ( 1.000000000000000000, 0.000000000000000000, -1.047444401652940007E-14 ) ) ;
#29456=CARTESIAN_POINT ( 'NONE',  ( 68.00000000000004263, -0.5000000000000000000, 1.988246715072644166 ) ) ;
#29474=EDGE_LOOP ( 'NONE', ( #21118, #13609 ) ) ;
#29503=ORIENTED_EDGE ( 'NONE', *, *, #30957, .F. ) ;
#29506=EDGE_CURVE ( 'NONE', #16699, #13465, #3883, .T. ) ;
#29519=VERTEX_POINT ( 'NONE', #7906 ) ;
#29543=FACE_OUTER_BOUND ( 'NONE', #22300, .T. ) ;
#29556=DIRECTION ( 'NONE',  ( 1.000000000000000000, 0.000000000000000000, -1.047444401652940007E-14 ) ) ;
#29558=AXIS2_PLACEMENT_3D ( 'NONE', #25827, #28215, #23457 ) ;
#29570=CIRCLE ( 'NONE', #12373, 0.05000000000000007216 ) ;
#29583=ORIENTED_EDGE ( 'NONE', *, *, #7513, .T. ) ;
#29595=DIRECTION ( 'NONE',  ( 0.000000000000000000, 0.000000000000000000, -1.000000000000000000 ) ) ;
#29596=CARTESIAN_POINT ( 'NONE',  ( 69.20000000000003126, 5.529431079676072613E-15, -7.248315259438346108E-13 ) ) ;
#29622=VERTEX_POINT ( 'NONE', #23269 ) ;
#29625=AXIS2_PLACEMENT_3D ( 'NONE', #5456, #12716, #22097 ) ;
#29666=CARTESIAN_POINT ( 'NONE',  ( 68.00000000000000000, -0.7500000000000000000, -1.988246715074068582 ) ) ;
#29678=CIRCLE ( 'NONE', #16032, 3.000000000000000000 ) ;
#29705=DIRECTION ( 'NONE',  ( 1.047444401652940007E-14, 0.000000000000000000, 1.000000000000000000 ) ) ;
#29727=DIRECTION ( 'NONE',  ( 7.401486830834377462E-15, 0.000000000000000000, 1.000000000000000000 ) ) ;
#29728=CARTESIAN_POINT ( 'NONE',  ( 65.00000000000002842, 1.401298464324817071E-42, -6.808388610744111684E-13 ) ) ;
#29753=DIRECTION ( 'NONE',  ( -3.696862594069181415E-15, -0.9356455129756988676, -0.3529411764705864263 ) ) ;
#29773=DIRECTION ( 'NONE',  ( 0.000000000000000000, 0.000000000000000000, -1.000000000000000000 ) ) ;
#29823=EDGE_CURVE ( 'NONE', #29022, #590, #22621, .T. ) ;
#29845=ADVANCED_FACE ( 'NONE', ( #19623 ), #2377, .T. ) ;
#29858=DIRECTION ( 'NONE',  ( 1.047444401652940007E-14, 0.000000000000000000, 1.000000000000000000 ) ) ;
#29862=DIRECTION ( 'NONE',  ( -1.000000000000000000, 0.000000000000000000, 1.047444401652940007E-14 ) ) ;
#29883=CARTESIAN_POINT ( 'NONE',  ( 68.00000000000001421, 3.252606517456513302E-16, -7.122621931239992550E-13 ) ) ;
#29900=FACE_OUTER_BOUND ( 'NONE', #13984, .T. ) ;
#29947=DIRECTION ( 'NONE',  ( 1.000000000000000000, -0.000000000000000000, -1.047444401652940007E-14 ) ) ;
#29982=FACE_OUTER_BOUND ( 'NONE', #16842, .T. ) ;
#29986=CIRCLE ( 'NONE', #7744, 2.624999999999998668 ) ;
#29990=ORIENTED_EDGE ( 'NONE', *, *, #26761, .F. ) ;
#29997=CARTESIAN_POINT ( 'NONE',  ( 69.25000000000001421, 5.529431079676072613E-15, -7.253552481446610839E-13 ) ) ;
#30011=DIRECTION ( 'NONE',  ( 1.282749433769087582E-30, 1.000000000000000000, 1.224646799147353207E-16 ) ) ;
#30025=CARTESIAN_POINT ( 'NONE',  ( 63.50000000000005684, 1.401298464324817071E-42, 2.624999999999333422 ) ) ;
#30027=CARTESIAN_POINT ( 'NONE',  ( 59.00000000000002132, 1.401298464324817071E-42, -6.179921969752347932E-13 ) ) ;
#30030=ORIENTED_EDGE ( 'NONE', *, *, #1766, .T. ) ;
#30031=CIRCLE ( 'NONE', #17906, 0.2500000000000000000 ) ;
#30044=CIRCLE ( 'NONE', #6803, 0.2500000000000000000 ) ;
#30051=CARTESIAN_POINT ( 'NONE',  ( 69.20000000000000284, 0.8558823529411767606, -2.268940368966791077 ) ) ;
#30085=DIRECTION ( 'NONE',  ( -1.047444401652940007E-14, 0.000000000000000000, -1.000000000000000000 ) ) ;
#30107=DIRECTION ( 'NONE',  ( -1.047444401652940007E-14, 0.000000000000000000, -1.000000000000000000 ) ) ;
#30133=AXIS2_PLACEMENT_3D ( 'NONE', #19528, #29174, #506 ) ;
#30160=AXIS2_PLACEMENT_3D ( 'NONE', #10804, #13485, #15576 ) ;
#30182=ORIENTED_EDGE ( 'NONE', *, *, #27509, .T. ) ;
#30190=AXIS2_PLACEMENT_3D ( 'NONE', #24810, #10247, #7864 ) ;
#30194=DIRECTION ( 'NONE',  ( 1.000000000000000000, 0.000000000000000000, -1.047444401652940007E-14 ) ) ;
#30208=ORIENTED_EDGE ( 'NONE', *, *, #8941, .T. ) ;
#30221=AXIS2_PLACEMENT_3D ( 'NONE', #4843, #15124, #25250 ) ;
#30255=ORIENTED_EDGE ( 'NONE', *, *, #11598, .T. ) ;
#30359=DIRECTION ( 'NONE',  ( 1.054009200593503061E-14, 0.000000000000000000, 1.000000000000000000 ) ) ;
#30369=ORIENTED_EDGE ( 'NONE', *, *, #10974, .F. ) ;
#30370=CARTESIAN_POINT ( 'NONE',  ( 63.50000000000000000, -0.7500000000000000000, -1.988246715074021731 ) ) ;
#30383=VERTEX_POINT ( 'NONE', #24359 ) ;
#30400=ORIENTED_EDGE ( 'NONE', *, *, #30535, .T. ) ;
#30401=AXIS2_PLACEMENT_3D ( 'NONE', #1340, #25881, #30462 ) ;
#30404=DIRECTION ( 'NONE',  ( -1.047444401652940007E-14, -8.673617379884032317E-15, -1.000000000000000000 ) ) ;
#30424=AXIS2_PLACEMENT_3D ( 'NONE', #28007, #1566, #6970 ) ;
#30430=CARTESIAN_POINT ( 'NONE',  ( 69.20000000000003126, 1.401298464324817071E-42, -7.248315259438346108E-13 ) ) ;
#30435=CARTESIAN_POINT ( 'NONE',  ( 59.00000000000002132, 1.401298464324817071E-42, -6.179921969752347932E-13 ) ) ;
#30462=DIRECTION ( 'NONE',  ( 1.047444401652940007E-14, 0.000000000000000000, 1.000000000000000000 ) ) ;
#30471=DIRECTION ( 'NONE',  ( -1.047444401652940007E-14, 0.000000000000000000, -1.000000000000000000 ) ) ;
#30478=ORIENTED_EDGE ( 'NONE', *, *, #6158, .F. ) ;
#30496=ORIENTED_EDGE ( 'NONE', *, *, #18817, .F. ) ;
#30521=ORIENTED_EDGE ( 'NONE', *, *, #8821, .F. ) ;
#30535=EDGE_CURVE ( 'NONE', #27508, #14261, #15555, .T. ) ;
#30539=VERTEX_POINT ( 'NONE', #8042 ) ;
#30557=DIRECTION ( 'NONE',  ( -1.000000000000000000, 0.000000000000000000, 1.047444401652940007E-14 ) ) ;
#30595=CARTESIAN_POINT ( 'NONE',  ( 49.04999999999999716, 1.401298464324817071E-42, -2.875000000000512923 ) ) ;
#30602=FACE_OUTER_BOUND ( 'NONE', #1517, .T. ) ;
#30619=EDGE_CURVE ( 'NONE', #14261, #7542, #25695, .T. ) ;
#30668=AXIS2_PLACEMENT_3D ( 'NONE', #22980, #13446, #13001 ) ;
#30689=ORIENTED_EDGE ( 'NONE', *, *, #15153, .F. ) ;
#30734=AXIS2_PLACEMENT_3D ( 'NONE', #4471, #7015, #14124 ) ;
#30738=EDGE_CURVE ( 'NONE', #28523, #171, #24679, .T. ) ;
#30775=EDGE_CURVE ( 'NONE', #5953, #5818, #22670, .T. ) ;
#30787=ORIENTED_EDGE ( 'NONE', *, *, #19982, .F. ) ;
#30806=LINE ( 'NONE', #26214, #22655 ) ;
#30825=ORIENTED_EDGE ( 'NONE', *, *, #20997, .T. ) ;
#30845=DIRECTION ( 'NONE',  ( -9.654113257610060303E-15, 0.000000000000000000, -1.000000000000000000 ) ) ;
#30850=EDGE_CURVE ( 'NONE', #29022, #27662, #6754, .T. ) ;
#30866=CARTESIAN_POINT ( 'NONE',  ( 63.50000000000002842, 1.401298464324817071E-42, -6.651271950496169736E-13 ) ) ;
#30867=CARTESIAN_POINT ( 'NONE',  ( 67.99999999999998579, 4.286263797015756316E-16, -3.500000000000712763 ) ) ;
#30868=CARTESIAN_POINT ( 'NONE',  ( 69.01464466094073202, 4.557543281186736018E-17, 2.985355339058589852 ) ) ;
#30885=DIRECTION ( 'NONE',  ( -1.000000000000000000, 0.000000000000000000, 1.047444401652940007E-14 ) ) ;
#30945=CARTESIAN_POINT ( 'NONE',  ( 63.50000000000002842, 1.401298464324817071E-42, -6.651271950496169736E-13 ) ) ;
#30957=EDGE_CURVE ( 'NONE', #15234, #5901, #9542, .T. ) ;
#30963=PLANE ( 'NONE',  #25163 ) ;
#30986=CYLINDRICAL_SURFACE ( 'NONE', #2376, 3.500000000000000444 ) ;
#30989=CARTESIAN_POINT ( 'NONE',  ( 69.20000000000004547, -0.5000000000000000000, 1.988246715072633508 ) ) ;
#31013=DIRECTION ( 'NONE',  ( 1.000000000000000000, -0.000000000000000000, -1.047444401652940007E-14 ) ) ;
#31054=VERTEX_POINT ( 'NONE', #18768 ) ;
#31058=CARTESIAN_POINT ( 'NONE',  ( 49.05000000000002558, 1.401298464324817071E-42, -5.137714790107672405E-13 ) ) ;
#31059=CIRCLE ( 'NONE', #3264, 0.2500000000000000000 ) ;
#31083=ADVANCED_FACE ( 'NONE', ( #11784 ), #23980, .F. ) ;
#31116=ORIENTED_EDGE ( 'NONE', *, *, #460, .F. ) ;
#31131=ORIENTED_EDGE ( 'NONE', *, *, #18929, .T. ) ;
#31134=AXIS2_PLACEMENT_3D ( 'NONE', #21446, #7035, #7334 ) ;
#31144=CIRCLE ( 'NONE', #9926, 0.04999999999999969746 ) ;
#31164=EDGE_CURVE ( 'NONE', #22848, #26053, #24219, .T. ) ;
#31176=DIRECTION ( 'NONE',  ( 1.000000000000000000, 0.000000000000000000, -1.047444401652940007E-14 ) ) ;
#31177=DIRECTION ( 'NONE',  ( -1.040834085586084257E-14, 0.000000000000000000, -1.000000000000000000 ) ) ;
#31227=VERTEX_POINT ( 'NONE', #24893 ) ;
#31228=CIRCLE ( 'NONE', #5436, 1.875000000000000000 ) ;
#31231=AXIS2_PLACEMENT_3D ( 'NONE', #26425, #31013, #12029 ) ;
#31250=CARTESIAN_POINT ( 'NONE',  ( 69.25000000000004263, 0.4500000000000000111, 1.988246715072633508 ) ) ;
#31265=ORIENTED_EDGE ( 'NONE', *, *, #19184, .F. ) ;
#31285=ADVANCED_FACE ( 'NONE', ( #15395 ), #937, .T. ) ;
#31289=CARTESIAN_POINT ( 'NONE',  ( 69.25000000000000000, -0.4500000000000000111, -1.988246715074081905 ) ) ;
#31290=VERTEX_POINT ( 'NONE', #8125 ) ;
#31299=EDGE_CURVE ( 'NONE', #12273, #4809, #27727, .T. ) ;
#31304=CARTESIAN_POINT ( 'NONE',  ( 49.00000000000002132, 1.401298464324817071E-42, -5.132477568099407673E-13 ) ) ;
#31308=DIRECTION ( 'NONE',  ( 9.824982518806699669E-15, 0.000000000000000000, 1.000000000000000000 ) ) ;
ENDSEC;
END-ISO-10303-21;
